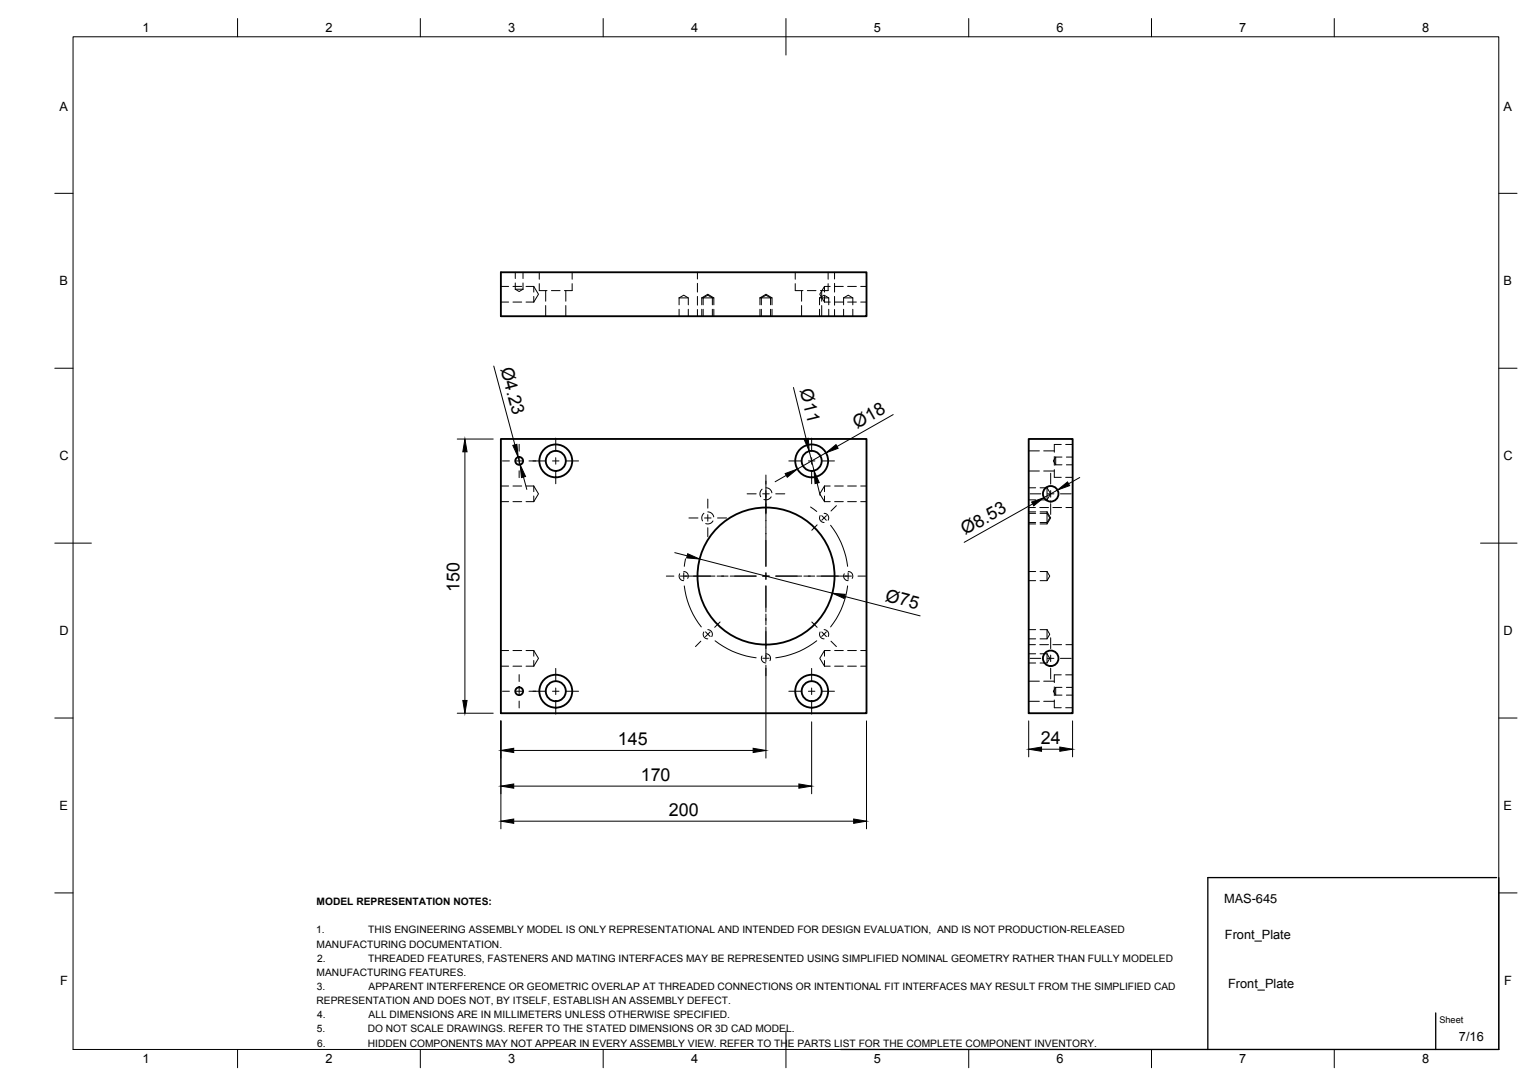
ISO-10303-21;
HEADER;
FILE_DESCRIPTION((''),'2;1');
FILE_NAME('Front_Plate.step','2026-10-09T10:54:55-07:00',(''),(''),'','','');
FILE_SCHEMA (('AUTOMOTIVE_DESIGN { 1 0 10303 214 3 1 1 }'));
ENDSEC;
DATA;
#10=MECHANICAL_DESIGN_GEOMETRIC_PRESENTATION_REPRESENTATION('',(#598),#63824);
#568=SHAPE_REPRESENTATION_RELATIONSHIP('SRR','None',#63882,#583) ;
#583=ADVANCED_BREP_SHAPE_REPRESENTATION('',(#613),#63812) ;
#598=STYLED_ITEM('',(#63963),#613) ;
#613=MANIFOLD_SOLID_BREP('Body1',#15497) ;
#695=FACE_BOUND('',#2596,.T.) ;
#696=FACE_BOUND('',#2600,.T.) ;
#697=FACE_BOUND('',#2604,.T.) ;
#698=FACE_BOUND('',#2608,.T.) ;
#699=FACE_BOUND('',#2629,.T.) ;
#700=FACE_BOUND('',#2630,.T.) ;
#701=FACE_BOUND('',#2633,.T.) ;
#702=FACE_BOUND('',#2634,.T.) ;
#703=FACE_BOUND('',#2637,.T.) ;
#704=FACE_BOUND('',#2638,.T.) ;
#705=FACE_BOUND('',#2639,.T.) ;
#706=FACE_BOUND('',#2640,.T.) ;
#707=FACE_BOUND('',#2641,.T.) ;
#708=FACE_BOUND('',#2642,.T.) ;
#709=FACE_BOUND('',#2643,.T.) ;
#710=FACE_BOUND('',#2645,.T.) ;
#711=FACE_BOUND('',#2646,.T.) ;
#712=FACE_BOUND('',#2647,.T.) ;
#713=FACE_BOUND('',#2648,.T.) ;
#714=FACE_BOUND('',#2649,.T.) ;
#715=FACE_BOUND('',#2650,.T.) ;
#716=FACE_BOUND('',#2651,.T.) ;
#717=FACE_BOUND('',#2652,.T.) ;
#718=FACE_BOUND('',#2653,.T.) ;
#719=FACE_BOUND('',#2654,.T.) ;
#720=FACE_BOUND('',#2655,.T.) ;
#721=FACE_BOUND('',#2656,.T.) ;
#722=FACE_BOUND('',#2657,.T.) ;
#866=PLANE('',#15917) ;
#867=PLANE('',#15924) ;
#868=PLANE('',#15931) ;
#869=PLANE('',#15938) ;
#870=PLANE('',#15980) ;
#871=PLANE('',#15981) ;
#872=PLANE('',#15982) ;
#873=PLANE('',#15983) ;
#874=PLANE('',#15984) ;
#875=PLANE('',#15985) ;
#1169=CYLINDRICAL_SURFACE('',#15895,2.117) ;
#1170=CYLINDRICAL_SURFACE('',#15899,2.117) ;
#1171=CYLINDRICAL_SURFACE('',#15903,4.263) ;
#1172=CYLINDRICAL_SURFACE('',#15907,4.263) ;
#1173=CYLINDRICAL_SURFACE('',#15911,4.263) ;
#1174=CYLINDRICAL_SURFACE('',#15915,4.263) ;
#1175=CYLINDRICAL_SURFACE('',#15920,9.) ;
#1176=CYLINDRICAL_SURFACE('',#15922,5.5) ;
#1177=CYLINDRICAL_SURFACE('',#15927,9.) ;
#1178=CYLINDRICAL_SURFACE('',#15929,5.5) ;
#1179=CYLINDRICAL_SURFACE('',#15934,9.) ;
#1180=CYLINDRICAL_SURFACE('',#15936,5.5) ;
#1181=CYLINDRICAL_SURFACE('',#15941,9.) ;
#1182=CYLINDRICAL_SURFACE('',#15943,5.5) ;
#1183=CYLINDRICAL_SURFACE('',#15947,3.3) ;
#1184=CYLINDRICAL_SURFACE('',#15951,2.5175) ;
#1185=CYLINDRICAL_SURFACE('',#15955,2.5175) ;
#1186=CYLINDRICAL_SURFACE('',#15959,2.5175) ;
#1187=CYLINDRICAL_SURFACE('',#15963,2.5175) ;
#1188=CYLINDRICAL_SURFACE('',#15967,2.5175) ;
#1189=CYLINDRICAL_SURFACE('',#15971,2.5175) ;
#1190=CYLINDRICAL_SURFACE('',#15975,3.3) ;
#1191=CYLINDRICAL_SURFACE('',#15977,37.5) ;
#1652=FACE_OUTER_BOUND('',#2583,.T.) ;
#1653=FACE_OUTER_BOUND('',#2584,.T.) ;
#1654=FACE_OUTER_BOUND('',#2585,.T.) ;
#1655=FACE_OUTER_BOUND('',#2586,.T.) ;
#1656=FACE_OUTER_BOUND('',#2587,.T.) ;
#1657=FACE_OUTER_BOUND('',#2588,.T.) ;
#1658=FACE_OUTER_BOUND('',#2589,.T.) ;
#1659=FACE_OUTER_BOUND('',#2590,.T.) ;
#1660=FACE_OUTER_BOUND('',#2591,.T.) ;
#1661=FACE_OUTER_BOUND('',#2592,.T.) ;
#1662=FACE_OUTER_BOUND('',#2593,.T.) ;
#1663=FACE_OUTER_BOUND('',#2594,.T.) ;
#1664=FACE_OUTER_BOUND('',#2595,.T.) ;
#1665=FACE_OUTER_BOUND('',#2597,.T.) ;
#1666=FACE_OUTER_BOUND('',#2598,.T.) ;
#1667=FACE_OUTER_BOUND('',#2599,.T.) ;
#1668=FACE_OUTER_BOUND('',#2601,.T.) ;
#1669=FACE_OUTER_BOUND('',#2602,.T.) ;
#1670=FACE_OUTER_BOUND('',#2603,.T.) ;
#1671=FACE_OUTER_BOUND('',#2605,.T.) ;
#1672=FACE_OUTER_BOUND('',#2606,.T.) ;
#1673=FACE_OUTER_BOUND('',#2607,.T.) ;
#1674=FACE_OUTER_BOUND('',#2609,.T.) ;
#1675=FACE_OUTER_BOUND('',#2610,.T.) ;
#1676=FACE_OUTER_BOUND('',#2611,.T.) ;
#1677=FACE_OUTER_BOUND('',#2612,.T.) ;
#1678=FACE_OUTER_BOUND('',#2613,.T.) ;
#1679=FACE_OUTER_BOUND('',#2614,.T.) ;
#1680=FACE_OUTER_BOUND('',#2615,.T.) ;
#1681=FACE_OUTER_BOUND('',#2616,.T.) ;
#1682=FACE_OUTER_BOUND('',#2617,.T.) ;
#1683=FACE_OUTER_BOUND('',#2618,.T.) ;
#1684=FACE_OUTER_BOUND('',#2619,.T.) ;
#1685=FACE_OUTER_BOUND('',#2620,.T.) ;
#1686=FACE_OUTER_BOUND('',#2621,.T.) ;
#1687=FACE_OUTER_BOUND('',#2622,.T.) ;
#1688=FACE_OUTER_BOUND('',#2623,.T.) ;
#1689=FACE_OUTER_BOUND('',#2624,.T.) ;
#1690=FACE_OUTER_BOUND('',#2625,.T.) ;
#1691=FACE_OUTER_BOUND('',#2626,.T.) ;
#1692=FACE_OUTER_BOUND('',#2627,.T.) ;
#1693=FACE_OUTER_BOUND('',#2628,.T.) ;
#1694=FACE_OUTER_BOUND('',#2631,.T.) ;
#1695=FACE_OUTER_BOUND('',#2632,.T.) ;
#1696=FACE_OUTER_BOUND('',#2635,.T.) ;
#1697=FACE_OUTER_BOUND('',#2636,.T.) ;
#1698=FACE_OUTER_BOUND('',#2644,.T.) ;
#2583=EDGE_LOOP('',(#10232,#10233,#10234)) ;
#2584=EDGE_LOOP('',(#10235,#10236,#10237,#10238)) ;
#2585=EDGE_LOOP('',(#10239,#10240,#10241)) ;
#2586=EDGE_LOOP('',(#10242,#10243,#10244,#10245)) ;
#2587=EDGE_LOOP('',(#10246,#10247,#10248)) ;
#2588=EDGE_LOOP('',(#10249,#10250,#10251,#10252)) ;
#2589=EDGE_LOOP('',(#10253,#10254,#10255)) ;
#2590=EDGE_LOOP('',(#10256,#10257,#10258,#10259)) ;
#2591=EDGE_LOOP('',(#10260,#10261,#10262)) ;
#2592=EDGE_LOOP('',(#10263,#10264,#10265,#10266)) ;
#2593=EDGE_LOOP('',(#10267,#10268,#10269)) ;
#2594=EDGE_LOOP('',(#10270,#10271,#10272,#10273)) ;
#2595=EDGE_LOOP('',(#10274)) ;
#2596=EDGE_LOOP('',(#10275)) ;
#2597=EDGE_LOOP('',(#10276,#10277,#10278,#10279)) ;
#2598=EDGE_LOOP('',(#10280,#10281,#10282,#10283)) ;
#2599=EDGE_LOOP('',(#10284)) ;
#2600=EDGE_LOOP('',(#10285)) ;
#2601=EDGE_LOOP('',(#10286,#10287,#10288,#10289)) ;
#2602=EDGE_LOOP('',(#10290,#10291,#10292,#10293)) ;
#2603=EDGE_LOOP('',(#10294)) ;
#2604=EDGE_LOOP('',(#10295)) ;
#2605=EDGE_LOOP('',(#10296,#10297,#10298,#10299)) ;
#2606=EDGE_LOOP('',(#10300,#10301,#10302,#10303)) ;
#2607=EDGE_LOOP('',(#10304)) ;
#2608=EDGE_LOOP('',(#10305)) ;
#2609=EDGE_LOOP('',(#10306,#10307,#10308,#10309)) ;
#2610=EDGE_LOOP('',(#10310,#10311,#10312,#10313)) ;
#2611=EDGE_LOOP('',(#10314,#10315,#10316)) ;
#2612=EDGE_LOOP('',(#10317,#10318,#10319,#10320)) ;
#2613=EDGE_LOOP('',(#10321,#10322,#10323)) ;
#2614=EDGE_LOOP('',(#10324,#10325,#10326,#10327)) ;
#2615=EDGE_LOOP('',(#10328,#10329,#10330)) ;
#2616=EDGE_LOOP('',(#10331,#10332,#10333,#10334)) ;
#2617=EDGE_LOOP('',(#10335,#10336,#10337)) ;
#2618=EDGE_LOOP('',(#10338,#10339,#10340,#10341)) ;
#2619=EDGE_LOOP('',(#10342,#10343,#10344)) ;
#2620=EDGE_LOOP('',(#10345,#10346,#10347,#10348)) ;
#2621=EDGE_LOOP('',(#10349,#10350,#10351)) ;
#2622=EDGE_LOOP('',(#10352,#10353,#10354,#10355)) ;
#2623=EDGE_LOOP('',(#10356,#10357,#10358)) ;
#2624=EDGE_LOOP('',(#10359,#10360,#10361,#10362)) ;
#2625=EDGE_LOOP('',(#10363,#10364,#10365)) ;
#2626=EDGE_LOOP('',(#10366,#10367,#10368,#10369)) ;
#2627=EDGE_LOOP('',(#10370,#10371,#10372,#10373)) ;
#2628=EDGE_LOOP('',(#10374,#10375,#10376,#10377)) ;
#2629=EDGE_LOOP('',(#10378)) ;
#2630=EDGE_LOOP('',(#10379)) ;
#2631=EDGE_LOOP('',(#10380,#10381,#10382,#10383)) ;
#2632=EDGE_LOOP('',(#10384,#10385,#10386,#10387)) ;
#2633=EDGE_LOOP('',(#10388)) ;
#2634=EDGE_LOOP('',(#10389)) ;
#2635=EDGE_LOOP('',(#10390,#10391,#10392,#10393)) ;
#2636=EDGE_LOOP('',(#10394,#10395,#10396,#10397)) ;
#2637=EDGE_LOOP('',(#10398)) ;
#2638=EDGE_LOOP('',(#10399)) ;
#2639=EDGE_LOOP('',(#10400)) ;
#2640=EDGE_LOOP('',(#10401)) ;
#2641=EDGE_LOOP('',(#10402)) ;
#2642=EDGE_LOOP('',(#10403)) ;
#2643=EDGE_LOOP('',(#10404)) ;
#2644=EDGE_LOOP('',(#10405,#10406,#10407,#10408)) ;
#2645=EDGE_LOOP('',(#10409)) ;
#2646=EDGE_LOOP('',(#10410)) ;
#2647=EDGE_LOOP('',(#10411)) ;
#2648=EDGE_LOOP('',(#10412)) ;
#2649=EDGE_LOOP('',(#10413)) ;
#2650=EDGE_LOOP('',(#10414)) ;
#2651=EDGE_LOOP('',(#10415)) ;
#2652=EDGE_LOOP('',(#10416)) ;
#2653=EDGE_LOOP('',(#10417)) ;
#2654=EDGE_LOOP('',(#10418)) ;
#2655=EDGE_LOOP('',(#10419)) ;
#2656=EDGE_LOOP('',(#10420)) ;
#2657=EDGE_LOOP('',(#10421)) ;
#3580=CIRCLE('',#15894,2.117) ;
#3581=CIRCLE('',#15896,2.117) ;
#3582=CIRCLE('',#15898,2.117) ;
#3583=CIRCLE('',#15900,2.117) ;
#3584=CIRCLE('',#15902,4.263) ;
#3585=CIRCLE('',#15904,4.263) ;
#3586=CIRCLE('',#15906,4.263) ;
#3587=CIRCLE('',#15908,4.263) ;
#3588=CIRCLE('',#15910,4.263) ;
#3589=CIRCLE('',#15912,4.263) ;
#3590=CIRCLE('',#15914,4.263) ;
#3591=CIRCLE('',#15916,4.263) ;
#3592=CIRCLE('',#15918,9.) ;
#3593=CIRCLE('',#15919,5.5) ;
#3594=CIRCLE('',#15921,9.) ;
#3595=CIRCLE('',#15923,5.5) ;
#3596=CIRCLE('',#15925,9.) ;
#3597=CIRCLE('',#15926,5.5) ;
#3598=CIRCLE('',#15928,9.) ;
#3599=CIRCLE('',#15930,5.5) ;
#3600=CIRCLE('',#15932,9.) ;
#3601=CIRCLE('',#15933,5.5) ;
#3602=CIRCLE('',#15935,9.) ;
#3603=CIRCLE('',#15937,5.5) ;
#3604=CIRCLE('',#15939,9.) ;
#3605=CIRCLE('',#15940,5.5) ;
#3606=CIRCLE('',#15942,9.) ;
#3607=CIRCLE('',#15944,5.5) ;
#3608=CIRCLE('',#15946,3.3) ;
#3609=CIRCLE('',#15948,3.3) ;
#3610=CIRCLE('',#15950,2.5175) ;
#3611=CIRCLE('',#15952,2.5175) ;
#3612=CIRCLE('',#15954,2.5175) ;
#3613=CIRCLE('',#15956,2.5175) ;
#3614=CIRCLE('',#15958,2.5175) ;
#3615=CIRCLE('',#15960,2.5175) ;
#3616=CIRCLE('',#15962,2.5175) ;
#3617=CIRCLE('',#15964,2.5175) ;
#3618=CIRCLE('',#15966,2.5175) ;
#3619=CIRCLE('',#15968,2.5175) ;
#3620=CIRCLE('',#15970,2.5175) ;
#3621=CIRCLE('',#15972,2.5175) ;
#3622=CIRCLE('',#15974,3.3) ;
#3623=CIRCLE('',#15976,3.3) ;
#3624=CIRCLE('',#15978,37.5) ;
#3625=CIRCLE('',#15979,37.5) ;
#4799=LINE('',#23492,#5455) ;
#4800=LINE('',#23497,#5456) ;
#4801=LINE('',#23501,#5457) ;
#4802=LINE('',#23506,#5458) ;
#4803=LINE('',#23510,#5459) ;
#4804=LINE('',#23515,#5460) ;
#4805=LINE('',#23519,#5461) ;
#4806=LINE('',#23524,#5462) ;
#4807=LINE('',#23528,#5463) ;
#4808=LINE('',#23533,#5464) ;
#4809=LINE('',#23537,#5465) ;
#4810=LINE('',#23542,#5466) ;
#4811=LINE('',#23550,#5467) ;
#4812=LINE('',#23555,#5468) ;
#4813=LINE('',#23563,#5469) ;
#4814=LINE('',#23568,#5470) ;
#4815=LINE('',#23576,#5471) ;
#4816=LINE('',#23581,#5472) ;
#4817=LINE('',#23589,#5473) ;
#4818=LINE('',#23594,#5474) ;
#4819=LINE('',#23598,#5475) ;
#4820=LINE('',#23602,#5476) ;
#4821=LINE('',#23607,#5477) ;
#4822=LINE('',#23611,#5478) ;
#4823=LINE('',#23616,#5479) ;
#4824=LINE('',#23620,#5480) ;
#4825=LINE('',#23625,#5481) ;
#4826=LINE('',#23629,#5482) ;
#4827=LINE('',#23634,#5483) ;
#4828=LINE('',#23638,#5484) ;
#4829=LINE('',#23643,#5485) ;
#4830=LINE('',#23647,#5486) ;
#4831=LINE('',#23652,#5487) ;
#4832=LINE('',#23656,#5488) ;
#4833=LINE('',#23661,#5489) ;
#4834=LINE('',#23665,#5490) ;
#4835=LINE('',#23671,#5491) ;
#4836=LINE('',#23676,#5492) ;
#4837=LINE('',#23678,#5493) ;
#4838=LINE('',#23680,#5494) ;
#4839=LINE('',#23681,#5495) ;
#4840=LINE('',#23684,#5496) ;
#4841=LINE('',#23686,#5497) ;
#4842=LINE('',#23687,#5498) ;
#4843=LINE('',#23690,#5499) ;
#4844=LINE('',#23692,#5500) ;
#4845=LINE('',#23693,#5501) ;
#4846=LINE('',#23695,#5502) ;
#4847=LINE('',#23696,#5503) ;
#5455=VECTOR('',#18449,1.20708774962173) ;
#5456=VECTOR('',#18456,2.117) ;
#5457=VECTOR('',#18459,1.20708774962173) ;
#5458=VECTOR('',#18466,2.117) ;
#5459=VECTOR('',#18469,2.42186816158307) ;
#5460=VECTOR('',#18476,4.263) ;
#5461=VECTOR('',#18479,2.42186816158307) ;
#5462=VECTOR('',#18486,4.263) ;
#5463=VECTOR('',#18489,2.42186816158307) ;
#5464=VECTOR('',#18496,4.263) ;
#5465=VECTOR('',#18499,2.42186816158307) ;
#5466=VECTOR('',#18506,4.263) ;
#5467=VECTOR('',#18515,9.) ;
#5468=VECTOR('',#18522,5.5) ;
#5469=VECTOR('',#18531,9.) ;
#5470=VECTOR('',#18538,5.5) ;
#5471=VECTOR('',#18547,9.) ;
#5472=VECTOR('',#18554,5.5) ;
#5473=VECTOR('',#18563,9.) ;
#5474=VECTOR('',#18570,5.5) ;
#5475=VECTOR('',#18573,1.65) ;
#5476=VECTOR('',#18578,3.3) ;
#5477=VECTOR('',#18583,1.44243074893998) ;
#5478=VECTOR('',#18588,2.5175) ;
#5479=VECTOR('',#18593,1.44243074893998) ;
#5480=VECTOR('',#18598,2.5175) ;
#5481=VECTOR('',#18603,1.44243074893998) ;
#5482=VECTOR('',#18608,2.5175) ;
#5483=VECTOR('',#18613,1.44243074893998) ;
#5484=VECTOR('',#18618,2.5175) ;
#5485=VECTOR('',#18623,1.44243074893998) ;
#5486=VECTOR('',#18628,2.5175) ;
#5487=VECTOR('',#18633,1.44243074893998) ;
#5488=VECTOR('',#18638,2.5175) ;
#5489=VECTOR('',#18643,1.65) ;
#5490=VECTOR('',#18648,3.3) ;
#5491=VECTOR('',#18655,37.5) ;
#5492=VECTOR('',#18660,10.) ;
#5493=VECTOR('',#18661,10.) ;
#5494=VECTOR('',#18662,10.) ;
#5495=VECTOR('',#18663,10.) ;
#5496=VECTOR('',#18666,10.) ;
#5497=VECTOR('',#18667,10.) ;
#5498=VECTOR('',#18668,10.) ;
#5499=VECTOR('',#18671,10.) ;
#5500=VECTOR('',#18672,10.) ;
#5501=VECTOR('',#18673,10.) ;
#5502=VECTOR('',#18676,10.) ;
#5503=VECTOR('',#18677,10.) ;
#6152=VERTEX_POINT('',#23490) ;
#6153=VERTEX_POINT('',#23491) ;
#6154=VERTEX_POINT('',#23495) ;
#6155=VERTEX_POINT('',#23499) ;
#6156=VERTEX_POINT('',#23500) ;
#6157=VERTEX_POINT('',#23504) ;
#6158=VERTEX_POINT('',#23508) ;
#6159=VERTEX_POINT('',#23509) ;
#6160=VERTEX_POINT('',#23513) ;
#6161=VERTEX_POINT('',#23517) ;
#6162=VERTEX_POINT('',#23518) ;
#6163=VERTEX_POINT('',#23522) ;
#6164=VERTEX_POINT('',#23526) ;
#6165=VERTEX_POINT('',#23527) ;
#6166=VERTEX_POINT('',#23531) ;
#6167=VERTEX_POINT('',#23535) ;
#6168=VERTEX_POINT('',#23536) ;
#6169=VERTEX_POINT('',#23540) ;
#6170=VERTEX_POINT('',#23544) ;
#6171=VERTEX_POINT('',#23546) ;
#6172=VERTEX_POINT('',#23549) ;
#6173=VERTEX_POINT('',#23553) ;
#6174=VERTEX_POINT('',#23557) ;
#6175=VERTEX_POINT('',#23559) ;
#6176=VERTEX_POINT('',#23562) ;
#6177=VERTEX_POINT('',#23566) ;
#6178=VERTEX_POINT('',#23570) ;
#6179=VERTEX_POINT('',#23572) ;
#6180=VERTEX_POINT('',#23575) ;
#6181=VERTEX_POINT('',#23579) ;
#6182=VERTEX_POINT('',#23583) ;
#6183=VERTEX_POINT('',#23585) ;
#6184=VERTEX_POINT('',#23588) ;
#6185=VERTEX_POINT('',#23592) ;
#6186=VERTEX_POINT('',#23596) ;
#6187=VERTEX_POINT('',#23597) ;
#6188=VERTEX_POINT('',#23601) ;
#6189=VERTEX_POINT('',#23605) ;
#6190=VERTEX_POINT('',#23606) ;
#6191=VERTEX_POINT('',#23610) ;
#6192=VERTEX_POINT('',#23614) ;
#6193=VERTEX_POINT('',#23615) ;
#6194=VERTEX_POINT('',#23619) ;
#6195=VERTEX_POINT('',#23623) ;
#6196=VERTEX_POINT('',#23624) ;
#6197=VERTEX_POINT('',#23628) ;
#6198=VERTEX_POINT('',#23632) ;
#6199=VERTEX_POINT('',#23633) ;
#6200=VERTEX_POINT('',#23637) ;
#6201=VERTEX_POINT('',#23641) ;
#6202=VERTEX_POINT('',#23642) ;
#6203=VERTEX_POINT('',#23646) ;
#6204=VERTEX_POINT('',#23650) ;
#6205=VERTEX_POINT('',#23651) ;
#6206=VERTEX_POINT('',#23655) ;
#6207=VERTEX_POINT('',#23659) ;
#6208=VERTEX_POINT('',#23660) ;
#6209=VERTEX_POINT('',#23664) ;
#6210=VERTEX_POINT('',#23668) ;
#6211=VERTEX_POINT('',#23670) ;
#6212=VERTEX_POINT('',#23674) ;
#6213=VERTEX_POINT('',#23675) ;
#6214=VERTEX_POINT('',#23677) ;
#6215=VERTEX_POINT('',#23679) ;
#6216=VERTEX_POINT('',#23683) ;
#6217=VERTEX_POINT('',#23685) ;
#6218=VERTEX_POINT('',#23689) ;
#6219=VERTEX_POINT('',#23691) ;
#7670=EDGE_CURVE('',#6152,#6153,#4799,.T.) ;
#7671=EDGE_CURVE('',#6153,#6153,#3580,.T.) ;
#7672=EDGE_CURVE('',#6154,#6154,#3581,.T.) ;
#7673=EDGE_CURVE('',#6154,#6153,#4800,.T.) ;
#7674=EDGE_CURVE('',#6155,#6156,#4801,.T.) ;
#7675=EDGE_CURVE('',#6156,#6156,#3582,.T.) ;
#7676=EDGE_CURVE('',#6157,#6157,#3583,.T.) ;
#7677=EDGE_CURVE('',#6157,#6156,#4802,.T.) ;
#7678=EDGE_CURVE('',#6158,#6159,#4803,.T.) ;
#7679=EDGE_CURVE('',#6159,#6159,#3584,.T.) ;
#7680=EDGE_CURVE('',#6160,#6160,#3585,.T.) ;
#7681=EDGE_CURVE('',#6160,#6159,#4804,.T.) ;
#7682=EDGE_CURVE('',#6161,#6162,#4805,.T.) ;
#7683=EDGE_CURVE('',#6162,#6162,#3586,.T.) ;
#7684=EDGE_CURVE('',#6163,#6163,#3587,.T.) ;
#7685=EDGE_CURVE('',#6163,#6162,#4806,.T.) ;
#7686=EDGE_CURVE('',#6164,#6165,#4807,.T.) ;
#7687=EDGE_CURVE('',#6165,#6165,#3588,.T.) ;
#7688=EDGE_CURVE('',#6166,#6166,#3589,.T.) ;
#7689=EDGE_CURVE('',#6166,#6165,#4808,.T.) ;
#7690=EDGE_CURVE('',#6167,#6168,#4809,.T.) ;
#7691=EDGE_CURVE('',#6168,#6168,#3590,.T.) ;
#7692=EDGE_CURVE('',#6169,#6169,#3591,.T.) ;
#7693=EDGE_CURVE('',#6169,#6168,#4810,.T.) ;
#7694=EDGE_CURVE('',#6170,#6170,#3592,.T.) ;
#7695=EDGE_CURVE('',#6171,#6171,#3593,.T.) ;
#7696=EDGE_CURVE('',#6170,#6172,#4811,.T.) ;
#7697=EDGE_CURVE('',#6172,#6172,#3594,.T.) ;
#7698=EDGE_CURVE('',#6173,#6173,#3595,.T.) ;
#7699=EDGE_CURVE('',#6173,#6171,#4812,.T.) ;
#7700=EDGE_CURVE('',#6174,#6174,#3596,.T.) ;
#7701=EDGE_CURVE('',#6175,#6175,#3597,.T.) ;
#7702=EDGE_CURVE('',#6174,#6176,#4813,.T.) ;
#7703=EDGE_CURVE('',#6176,#6176,#3598,.T.) ;
#7704=EDGE_CURVE('',#6177,#6177,#3599,.T.) ;
#7705=EDGE_CURVE('',#6177,#6175,#4814,.T.) ;
#7706=EDGE_CURVE('',#6178,#6178,#3600,.T.) ;
#7707=EDGE_CURVE('',#6179,#6179,#3601,.T.) ;
#7708=EDGE_CURVE('',#6178,#6180,#4815,.T.) ;
#7709=EDGE_CURVE('',#6180,#6180,#3602,.T.) ;
#7710=EDGE_CURVE('',#6181,#6181,#3603,.T.) ;
#7711=EDGE_CURVE('',#6181,#6179,#4816,.T.) ;
#7712=EDGE_CURVE('',#6182,#6182,#3604,.T.) ;
#7713=EDGE_CURVE('',#6183,#6183,#3605,.T.) ;
#7714=EDGE_CURVE('',#6182,#6184,#4817,.T.) ;
#7715=EDGE_CURVE('',#6184,#6184,#3606,.T.) ;
#7716=EDGE_CURVE('',#6185,#6185,#3607,.T.) ;
#7717=EDGE_CURVE('',#6185,#6183,#4818,.T.) ;
#7718=EDGE_CURVE('',#6186,#6187,#4819,.T.) ;
#7719=EDGE_CURVE('',#6187,#6187,#3608,.T.) ;
#7720=EDGE_CURVE('',#6187,#6188,#4820,.T.) ;
#7721=EDGE_CURVE('',#6188,#6188,#3609,.T.) ;
#7722=EDGE_CURVE('',#6189,#6190,#4821,.T.) ;
#7723=EDGE_CURVE('',#6190,#6190,#3610,.T.) ;
#7724=EDGE_CURVE('',#6190,#6191,#4822,.T.) ;
#7725=EDGE_CURVE('',#6191,#6191,#3611,.F.) ;
#7726=EDGE_CURVE('',#6192,#6193,#4823,.T.) ;
#7727=EDGE_CURVE('',#6193,#6193,#3612,.T.) ;
#7728=EDGE_CURVE('',#6193,#6194,#4824,.T.) ;
#7729=EDGE_CURVE('',#6194,#6194,#3613,.F.) ;
#7730=EDGE_CURVE('',#6195,#6196,#4825,.T.) ;
#7731=EDGE_CURVE('',#6196,#6196,#3614,.T.) ;
#7732=EDGE_CURVE('',#6196,#6197,#4826,.T.) ;
#7733=EDGE_CURVE('',#6197,#6197,#3615,.F.) ;
#7734=EDGE_CURVE('',#6198,#6199,#4827,.T.) ;
#7735=EDGE_CURVE('',#6199,#6199,#3616,.T.) ;
#7736=EDGE_CURVE('',#6199,#6200,#4828,.T.) ;
#7737=EDGE_CURVE('',#6200,#6200,#3617,.F.) ;
#7738=EDGE_CURVE('',#6201,#6202,#4829,.T.) ;
#7739=EDGE_CURVE('',#6202,#6202,#3618,.T.) ;
#7740=EDGE_CURVE('',#6202,#6203,#4830,.T.) ;
#7741=EDGE_CURVE('',#6203,#6203,#3619,.F.) ;
#7742=EDGE_CURVE('',#6204,#6205,#4831,.T.) ;
#7743=EDGE_CURVE('',#6205,#6205,#3620,.T.) ;
#7744=EDGE_CURVE('',#6205,#6206,#4832,.T.) ;
#7745=EDGE_CURVE('',#6206,#6206,#3621,.F.) ;
#7746=EDGE_CURVE('',#6207,#6208,#4833,.T.) ;
#7747=EDGE_CURVE('',#6208,#6208,#3622,.T.) ;
#7748=EDGE_CURVE('',#6208,#6209,#4834,.T.) ;
#7749=EDGE_CURVE('',#6209,#6209,#3623,.T.) ;
#7750=EDGE_CURVE('',#6210,#6210,#3624,.T.) ;
#7751=EDGE_CURVE('',#6210,#6211,#4835,.T.) ;
#7752=EDGE_CURVE('',#6211,#6211,#3625,.T.) ;
#7753=EDGE_CURVE('',#6212,#6213,#4836,.T.) ;
#7754=EDGE_CURVE('',#6213,#6214,#4837,.T.) ;
#7755=EDGE_CURVE('',#6214,#6215,#4838,.T.) ;
#7756=EDGE_CURVE('',#6212,#6215,#4839,.T.) ;
#7757=EDGE_CURVE('',#6213,#6216,#4840,.T.) ;
#7758=EDGE_CURVE('',#6216,#6217,#4841,.T.) ;
#7759=EDGE_CURVE('',#6217,#6214,#4842,.T.) ;
#7760=EDGE_CURVE('',#6218,#6216,#4843,.T.) ;
#7761=EDGE_CURVE('',#6218,#6219,#4844,.T.) ;
#7762=EDGE_CURVE('',#6219,#6217,#4845,.T.) ;
#7763=EDGE_CURVE('',#6218,#6212,#4846,.T.) ;
#7764=EDGE_CURVE('',#6215,#6219,#4847,.T.) ;
#10232=ORIENTED_EDGE('',*,*,#7670,.T.) ;
#10233=ORIENTED_EDGE('',*,*,#7671,.F.) ;
#10234=ORIENTED_EDGE('',*,*,#7670,.F.) ;
#10235=ORIENTED_EDGE('',*,*,#7672,.F.) ;
#10236=ORIENTED_EDGE('',*,*,#7673,.T.) ;
#10237=ORIENTED_EDGE('',*,*,#7671,.T.) ;
#10238=ORIENTED_EDGE('',*,*,#7673,.F.) ;
#10239=ORIENTED_EDGE('',*,*,#7674,.T.) ;
#10240=ORIENTED_EDGE('',*,*,#7675,.F.) ;
#10241=ORIENTED_EDGE('',*,*,#7674,.F.) ;
#10242=ORIENTED_EDGE('',*,*,#7676,.F.) ;
#10243=ORIENTED_EDGE('',*,*,#7677,.T.) ;
#10244=ORIENTED_EDGE('',*,*,#7675,.T.) ;
#10245=ORIENTED_EDGE('',*,*,#7677,.F.) ;
#10246=ORIENTED_EDGE('',*,*,#7678,.T.) ;
#10247=ORIENTED_EDGE('',*,*,#7679,.F.) ;
#10248=ORIENTED_EDGE('',*,*,#7678,.F.) ;
#10249=ORIENTED_EDGE('',*,*,#7680,.F.) ;
#10250=ORIENTED_EDGE('',*,*,#7681,.T.) ;
#10251=ORIENTED_EDGE('',*,*,#7679,.T.) ;
#10252=ORIENTED_EDGE('',*,*,#7681,.F.) ;
#10253=ORIENTED_EDGE('',*,*,#7682,.T.) ;
#10254=ORIENTED_EDGE('',*,*,#7683,.F.) ;
#10255=ORIENTED_EDGE('',*,*,#7682,.F.) ;
#10256=ORIENTED_EDGE('',*,*,#7684,.F.) ;
#10257=ORIENTED_EDGE('',*,*,#7685,.T.) ;
#10258=ORIENTED_EDGE('',*,*,#7683,.T.) ;
#10259=ORIENTED_EDGE('',*,*,#7685,.F.) ;
#10260=ORIENTED_EDGE('',*,*,#7686,.T.) ;
#10261=ORIENTED_EDGE('',*,*,#7687,.F.) ;
#10262=ORIENTED_EDGE('',*,*,#7686,.F.) ;
#10263=ORIENTED_EDGE('',*,*,#7688,.F.) ;
#10264=ORIENTED_EDGE('',*,*,#7689,.T.) ;
#10265=ORIENTED_EDGE('',*,*,#7687,.T.) ;
#10266=ORIENTED_EDGE('',*,*,#7689,.F.) ;
#10267=ORIENTED_EDGE('',*,*,#7690,.T.) ;
#10268=ORIENTED_EDGE('',*,*,#7691,.F.) ;
#10269=ORIENTED_EDGE('',*,*,#7690,.F.) ;
#10270=ORIENTED_EDGE('',*,*,#7692,.F.) ;
#10271=ORIENTED_EDGE('',*,*,#7693,.T.) ;
#10272=ORIENTED_EDGE('',*,*,#7691,.T.) ;
#10273=ORIENTED_EDGE('',*,*,#7693,.F.) ;
#10274=ORIENTED_EDGE('',*,*,#7694,.T.) ;
#10275=ORIENTED_EDGE('',*,*,#7695,.F.) ;
#10276=ORIENTED_EDGE('',*,*,#7694,.F.) ;
#10277=ORIENTED_EDGE('',*,*,#7696,.T.) ;
#10278=ORIENTED_EDGE('',*,*,#7697,.T.) ;
#10279=ORIENTED_EDGE('',*,*,#7696,.F.) ;
#10280=ORIENTED_EDGE('',*,*,#7698,.T.) ;
#10281=ORIENTED_EDGE('',*,*,#7699,.T.) ;
#10282=ORIENTED_EDGE('',*,*,#7695,.T.) ;
#10283=ORIENTED_EDGE('',*,*,#7699,.F.) ;
#10284=ORIENTED_EDGE('',*,*,#7700,.T.) ;
#10285=ORIENTED_EDGE('',*,*,#7701,.F.) ;
#10286=ORIENTED_EDGE('',*,*,#7700,.F.) ;
#10287=ORIENTED_EDGE('',*,*,#7702,.T.) ;
#10288=ORIENTED_EDGE('',*,*,#7703,.T.) ;
#10289=ORIENTED_EDGE('',*,*,#7702,.F.) ;
#10290=ORIENTED_EDGE('',*,*,#7704,.T.) ;
#10291=ORIENTED_EDGE('',*,*,#7705,.T.) ;
#10292=ORIENTED_EDGE('',*,*,#7701,.T.) ;
#10293=ORIENTED_EDGE('',*,*,#7705,.F.) ;
#10294=ORIENTED_EDGE('',*,*,#7706,.T.) ;
#10295=ORIENTED_EDGE('',*,*,#7707,.F.) ;
#10296=ORIENTED_EDGE('',*,*,#7706,.F.) ;
#10297=ORIENTED_EDGE('',*,*,#7708,.T.) ;
#10298=ORIENTED_EDGE('',*,*,#7709,.T.) ;
#10299=ORIENTED_EDGE('',*,*,#7708,.F.) ;
#10300=ORIENTED_EDGE('',*,*,#7710,.T.) ;
#10301=ORIENTED_EDGE('',*,*,#7711,.T.) ;
#10302=ORIENTED_EDGE('',*,*,#7707,.T.) ;
#10303=ORIENTED_EDGE('',*,*,#7711,.F.) ;
#10304=ORIENTED_EDGE('',*,*,#7712,.T.) ;
#10305=ORIENTED_EDGE('',*,*,#7713,.F.) ;
#10306=ORIENTED_EDGE('',*,*,#7712,.F.) ;
#10307=ORIENTED_EDGE('',*,*,#7714,.T.) ;
#10308=ORIENTED_EDGE('',*,*,#7715,.T.) ;
#10309=ORIENTED_EDGE('',*,*,#7714,.F.) ;
#10310=ORIENTED_EDGE('',*,*,#7716,.T.) ;
#10311=ORIENTED_EDGE('',*,*,#7717,.T.) ;
#10312=ORIENTED_EDGE('',*,*,#7713,.T.) ;
#10313=ORIENTED_EDGE('',*,*,#7717,.F.) ;
#10314=ORIENTED_EDGE('',*,*,#7718,.T.) ;
#10315=ORIENTED_EDGE('',*,*,#7719,.T.) ;
#10316=ORIENTED_EDGE('',*,*,#7718,.F.) ;
#10317=ORIENTED_EDGE('',*,*,#7719,.F.) ;
#10318=ORIENTED_EDGE('',*,*,#7720,.T.) ;
#10319=ORIENTED_EDGE('',*,*,#7721,.T.) ;
#10320=ORIENTED_EDGE('',*,*,#7720,.F.) ;
#10321=ORIENTED_EDGE('',*,*,#7722,.T.) ;
#10322=ORIENTED_EDGE('',*,*,#7723,.T.) ;
#10323=ORIENTED_EDGE('',*,*,#7722,.F.) ;
#10324=ORIENTED_EDGE('',*,*,#7723,.F.) ;
#10325=ORIENTED_EDGE('',*,*,#7724,.T.) ;
#10326=ORIENTED_EDGE('',*,*,#7725,.T.) ;
#10327=ORIENTED_EDGE('',*,*,#7724,.F.) ;
#10328=ORIENTED_EDGE('',*,*,#7726,.T.) ;
#10329=ORIENTED_EDGE('',*,*,#7727,.T.) ;
#10330=ORIENTED_EDGE('',*,*,#7726,.F.) ;
#10331=ORIENTED_EDGE('',*,*,#7727,.F.) ;
#10332=ORIENTED_EDGE('',*,*,#7728,.T.) ;
#10333=ORIENTED_EDGE('',*,*,#7729,.T.) ;
#10334=ORIENTED_EDGE('',*,*,#7728,.F.) ;
#10335=ORIENTED_EDGE('',*,*,#7730,.T.) ;
#10336=ORIENTED_EDGE('',*,*,#7731,.T.) ;
#10337=ORIENTED_EDGE('',*,*,#7730,.F.) ;
#10338=ORIENTED_EDGE('',*,*,#7731,.F.) ;
#10339=ORIENTED_EDGE('',*,*,#7732,.T.) ;
#10340=ORIENTED_EDGE('',*,*,#7733,.T.) ;
#10341=ORIENTED_EDGE('',*,*,#7732,.F.) ;
#10342=ORIENTED_EDGE('',*,*,#7734,.T.) ;
#10343=ORIENTED_EDGE('',*,*,#7735,.T.) ;
#10344=ORIENTED_EDGE('',*,*,#7734,.F.) ;
#10345=ORIENTED_EDGE('',*,*,#7735,.F.) ;
#10346=ORIENTED_EDGE('',*,*,#7736,.T.) ;
#10347=ORIENTED_EDGE('',*,*,#7737,.T.) ;
#10348=ORIENTED_EDGE('',*,*,#7736,.F.) ;
#10349=ORIENTED_EDGE('',*,*,#7738,.T.) ;
#10350=ORIENTED_EDGE('',*,*,#7739,.T.) ;
#10351=ORIENTED_EDGE('',*,*,#7738,.F.) ;
#10352=ORIENTED_EDGE('',*,*,#7739,.F.) ;
#10353=ORIENTED_EDGE('',*,*,#7740,.T.) ;
#10354=ORIENTED_EDGE('',*,*,#7741,.T.) ;
#10355=ORIENTED_EDGE('',*,*,#7740,.F.) ;
#10356=ORIENTED_EDGE('',*,*,#7742,.T.) ;
#10357=ORIENTED_EDGE('',*,*,#7743,.T.) ;
#10358=ORIENTED_EDGE('',*,*,#7742,.F.) ;
#10359=ORIENTED_EDGE('',*,*,#7743,.F.) ;
#10360=ORIENTED_EDGE('',*,*,#7744,.T.) ;
#10361=ORIENTED_EDGE('',*,*,#7745,.T.) ;
#10362=ORIENTED_EDGE('',*,*,#7744,.F.) ;
#10363=ORIENTED_EDGE('',*,*,#7746,.T.) ;
#10364=ORIENTED_EDGE('',*,*,#7747,.T.) ;
#10365=ORIENTED_EDGE('',*,*,#7746,.F.) ;
#10366=ORIENTED_EDGE('',*,*,#7747,.F.) ;
#10367=ORIENTED_EDGE('',*,*,#7748,.T.) ;
#10368=ORIENTED_EDGE('',*,*,#7749,.T.) ;
#10369=ORIENTED_EDGE('',*,*,#7748,.F.) ;
#10370=ORIENTED_EDGE('',*,*,#7750,.T.) ;
#10371=ORIENTED_EDGE('',*,*,#7751,.T.) ;
#10372=ORIENTED_EDGE('',*,*,#7752,.T.) ;
#10373=ORIENTED_EDGE('',*,*,#7751,.F.) ;
#10374=ORIENTED_EDGE('',*,*,#7753,.T.) ;
#10375=ORIENTED_EDGE('',*,*,#7754,.T.) ;
#10376=ORIENTED_EDGE('',*,*,#7755,.T.) ;
#10377=ORIENTED_EDGE('',*,*,#7756,.F.) ;
#10378=ORIENTED_EDGE('',*,*,#7688,.T.) ;
#10379=ORIENTED_EDGE('',*,*,#7692,.T.) ;
#10380=ORIENTED_EDGE('',*,*,#7757,.T.) ;
#10381=ORIENTED_EDGE('',*,*,#7758,.T.) ;
#10382=ORIENTED_EDGE('',*,*,#7759,.T.) ;
#10383=ORIENTED_EDGE('',*,*,#7754,.F.) ;
#10384=ORIENTED_EDGE('',*,*,#7760,.F.) ;
#10385=ORIENTED_EDGE('',*,*,#7761,.T.) ;
#10386=ORIENTED_EDGE('',*,*,#7762,.T.) ;
#10387=ORIENTED_EDGE('',*,*,#7758,.F.) ;
#10388=ORIENTED_EDGE('',*,*,#7680,.T.) ;
#10389=ORIENTED_EDGE('',*,*,#7684,.T.) ;
#10390=ORIENTED_EDGE('',*,*,#7763,.T.) ;
#10391=ORIENTED_EDGE('',*,*,#7756,.T.) ;
#10392=ORIENTED_EDGE('',*,*,#7764,.T.) ;
#10393=ORIENTED_EDGE('',*,*,#7761,.F.) ;
#10394=ORIENTED_EDGE('',*,*,#7763,.F.) ;
#10395=ORIENTED_EDGE('',*,*,#7760,.T.) ;
#10396=ORIENTED_EDGE('',*,*,#7757,.F.) ;
#10397=ORIENTED_EDGE('',*,*,#7753,.F.) ;
#10398=ORIENTED_EDGE('',*,*,#7672,.T.) ;
#10399=ORIENTED_EDGE('',*,*,#7676,.T.) ;
#10400=ORIENTED_EDGE('',*,*,#7697,.F.) ;
#10401=ORIENTED_EDGE('',*,*,#7703,.F.) ;
#10402=ORIENTED_EDGE('',*,*,#7709,.F.) ;
#10403=ORIENTED_EDGE('',*,*,#7715,.F.) ;
#10404=ORIENTED_EDGE('',*,*,#7752,.F.) ;
#10405=ORIENTED_EDGE('',*,*,#7764,.F.) ;
#10406=ORIENTED_EDGE('',*,*,#7755,.F.) ;
#10407=ORIENTED_EDGE('',*,*,#7759,.F.) ;
#10408=ORIENTED_EDGE('',*,*,#7762,.F.) ;
#10409=ORIENTED_EDGE('',*,*,#7698,.F.) ;
#10410=ORIENTED_EDGE('',*,*,#7704,.F.) ;
#10411=ORIENTED_EDGE('',*,*,#7710,.F.) ;
#10412=ORIENTED_EDGE('',*,*,#7716,.F.) ;
#10413=ORIENTED_EDGE('',*,*,#7721,.F.) ;
#10414=ORIENTED_EDGE('',*,*,#7725,.F.) ;
#10415=ORIENTED_EDGE('',*,*,#7729,.F.) ;
#10416=ORIENTED_EDGE('',*,*,#7733,.F.) ;
#10417=ORIENTED_EDGE('',*,*,#7737,.F.) ;
#10418=ORIENTED_EDGE('',*,*,#7741,.F.) ;
#10419=ORIENTED_EDGE('',*,*,#7745,.F.) ;
#10420=ORIENTED_EDGE('',*,*,#7749,.F.) ;
#10421=ORIENTED_EDGE('',*,*,#7750,.F.) ;
#14516=CONICAL_SURFACE('',#15893,1.20708774962173,1.02974425867665) ;
#14517=CONICAL_SURFACE('',#15897,1.20708774962173,1.02974425867665) ;
#14518=CONICAL_SURFACE('',#15901,2.42186816158307,1.02974425867665) ;
#14519=CONICAL_SURFACE('',#15905,2.42186816158307,1.02974425867665) ;
#14520=CONICAL_SURFACE('',#15909,2.42186816158307,1.02974425867665) ;
#14521=CONICAL_SURFACE('',#15913,2.42186816158307,1.02974425867665) ;
#14522=CONICAL_SURFACE('',#15945,1.65,1.02974425867665) ;
#14523=CONICAL_SURFACE('',#15949,1.44243074893998,1.02974425867665) ;
#14524=CONICAL_SURFACE('',#15953,1.44243074893998,1.02974425867665) ;
#14525=CONICAL_SURFACE('',#15957,1.44243074893998,1.02974425867665) ;
#14526=CONICAL_SURFACE('',#15961,1.44243074893998,1.02974425867665) ;
#14527=CONICAL_SURFACE('',#15965,1.44243074893998,1.02974425867665) ;
#14528=CONICAL_SURFACE('',#15969,1.44243074893998,1.02974425867665) ;
#14529=CONICAL_SURFACE('',#15973,1.65,1.02974425867665) ;
#14740=ADVANCED_FACE('',(#1652),#14516,.F.) ;
#14741=ADVANCED_FACE('',(#1653),#1169,.F.) ;
#14742=ADVANCED_FACE('',(#1654),#14517,.F.) ;
#14743=ADVANCED_FACE('',(#1655),#1170,.F.) ;
#14744=ADVANCED_FACE('',(#1656),#14518,.F.) ;
#14745=ADVANCED_FACE('',(#1657),#1171,.F.) ;
#14746=ADVANCED_FACE('',(#1658),#14519,.F.) ;
#14747=ADVANCED_FACE('',(#1659),#1172,.F.) ;
#14748=ADVANCED_FACE('',(#1660),#14520,.F.) ;
#14749=ADVANCED_FACE('',(#1661),#1173,.F.) ;
#14750=ADVANCED_FACE('',(#1662),#14521,.F.) ;
#14751=ADVANCED_FACE('',(#1663),#1174,.F.) ;
#14752=ADVANCED_FACE('',(#1664,#695),#866,.T.) ;
#14753=ADVANCED_FACE('',(#1665),#1175,.F.) ;
#14754=ADVANCED_FACE('',(#1666),#1176,.F.) ;
#14755=ADVANCED_FACE('',(#1667,#696),#867,.T.) ;
#14756=ADVANCED_FACE('',(#1668),#1177,.F.) ;
#14757=ADVANCED_FACE('',(#1669),#1178,.F.) ;
#14758=ADVANCED_FACE('',(#1670,#697),#868,.T.) ;
#14759=ADVANCED_FACE('',(#1671),#1179,.F.) ;
#14760=ADVANCED_FACE('',(#1672),#1180,.F.) ;
#14761=ADVANCED_FACE('',(#1673,#698),#869,.T.) ;
#14762=ADVANCED_FACE('',(#1674),#1181,.F.) ;
#14763=ADVANCED_FACE('',(#1675),#1182,.F.) ;
#14764=ADVANCED_FACE('',(#1676),#14522,.F.) ;
#14765=ADVANCED_FACE('',(#1677),#1183,.F.) ;
#14766=ADVANCED_FACE('',(#1678),#14523,.F.) ;
#14767=ADVANCED_FACE('',(#1679),#1184,.F.) ;
#14768=ADVANCED_FACE('',(#1680),#14524,.F.) ;
#14769=ADVANCED_FACE('',(#1681),#1185,.F.) ;
#14770=ADVANCED_FACE('',(#1682),#14525,.F.) ;
#14771=ADVANCED_FACE('',(#1683),#1186,.F.) ;
#14772=ADVANCED_FACE('',(#1684),#14526,.F.) ;
#14773=ADVANCED_FACE('',(#1685),#1187,.F.) ;
#14774=ADVANCED_FACE('',(#1686),#14527,.F.) ;
#14775=ADVANCED_FACE('',(#1687),#1188,.F.) ;
#14776=ADVANCED_FACE('',(#1688),#14528,.F.) ;
#14777=ADVANCED_FACE('',(#1689),#1189,.F.) ;
#14778=ADVANCED_FACE('',(#1690),#14529,.F.) ;
#14779=ADVANCED_FACE('',(#1691),#1190,.F.) ;
#14780=ADVANCED_FACE('',(#1692),#1191,.F.) ;
#14781=ADVANCED_FACE('',(#1693,#699,#700),#870,.F.) ;
#14782=ADVANCED_FACE('',(#1694),#871,.F.) ;
#14783=ADVANCED_FACE('',(#1695,#701,#702),#872,.F.) ;
#14784=ADVANCED_FACE('',(#1696),#873,.F.) ;
#14785=ADVANCED_FACE('',(#1697,#703,#704,#705,#706,#707,#708,#709),#874,
 .F.) ;
#14786=ADVANCED_FACE('',(#1698,#710,#711,#712,#713,#714,#715,#716,#717,
#718,#719,#720,#721,#722),#875,.T.) ;
#15497=CLOSED_SHELL('',(#14740,#14741,#14742,#14743,#14744,#14745,#14746,
#14747,#14748,#14749,#14750,#14751,#14752,#14753,#14754,#14755,#14756,#14757,
#14758,#14759,#14760,#14761,#14762,#14763,#14764,#14765,#14766,#14767,#14768,
#14769,#14770,#14771,#14772,#14773,#14774,#14775,#14776,#14777,#14778,#14779,
#14780,#14781,#14782,#14783,#14784,#14785,#14786)) ;
#15892=AXIS2_PLACEMENT_3D('',#23488,#18445,#18446) ;
#15893=AXIS2_PLACEMENT_3D('',#23489,#18447,#18448) ;
#15894=AXIS2_PLACEMENT_3D('',#23493,#18450,#18451) ;
#15895=AXIS2_PLACEMENT_3D('',#23494,#18452,#18453) ;
#15896=AXIS2_PLACEMENT_3D('',#23496,#18454,#18455) ;
#15897=AXIS2_PLACEMENT_3D('',#23498,#18457,#18458) ;
#15898=AXIS2_PLACEMENT_3D('',#23502,#18460,#18461) ;
#15899=AXIS2_PLACEMENT_3D('',#23503,#18462,#18463) ;
#15900=AXIS2_PLACEMENT_3D('',#23505,#18464,#18465) ;
#15901=AXIS2_PLACEMENT_3D('',#23507,#18467,#18468) ;
#15902=AXIS2_PLACEMENT_3D('',#23511,#18470,#18471) ;
#15903=AXIS2_PLACEMENT_3D('',#23512,#18472,#18473) ;
#15904=AXIS2_PLACEMENT_3D('',#23514,#18474,#18475) ;
#15905=AXIS2_PLACEMENT_3D('',#23516,#18477,#18478) ;
#15906=AXIS2_PLACEMENT_3D('',#23520,#18480,#18481) ;
#15907=AXIS2_PLACEMENT_3D('',#23521,#18482,#18483) ;
#15908=AXIS2_PLACEMENT_3D('',#23523,#18484,#18485) ;
#15909=AXIS2_PLACEMENT_3D('',#23525,#18487,#18488) ;
#15910=AXIS2_PLACEMENT_3D('',#23529,#18490,#18491) ;
#15911=AXIS2_PLACEMENT_3D('',#23530,#18492,#18493) ;
#15912=AXIS2_PLACEMENT_3D('',#23532,#18494,#18495) ;
#15913=AXIS2_PLACEMENT_3D('',#23534,#18497,#18498) ;
#15914=AXIS2_PLACEMENT_3D('',#23538,#18500,#18501) ;
#15915=AXIS2_PLACEMENT_3D('',#23539,#18502,#18503) ;
#15916=AXIS2_PLACEMENT_3D('',#23541,#18504,#18505) ;
#15917=AXIS2_PLACEMENT_3D('',#23543,#18507,#18508) ;
#15918=AXIS2_PLACEMENT_3D('',#23545,#18509,#18510) ;
#15919=AXIS2_PLACEMENT_3D('',#23547,#18511,#18512) ;
#15920=AXIS2_PLACEMENT_3D('',#23548,#18513,#18514) ;
#15921=AXIS2_PLACEMENT_3D('',#23551,#18516,#18517) ;
#15922=AXIS2_PLACEMENT_3D('',#23552,#18518,#18519) ;
#15923=AXIS2_PLACEMENT_3D('',#23554,#18520,#18521) ;
#15924=AXIS2_PLACEMENT_3D('',#23556,#18523,#18524) ;
#15925=AXIS2_PLACEMENT_3D('',#23558,#18525,#18526) ;
#15926=AXIS2_PLACEMENT_3D('',#23560,#18527,#18528) ;
#15927=AXIS2_PLACEMENT_3D('',#23561,#18529,#18530) ;
#15928=AXIS2_PLACEMENT_3D('',#23564,#18532,#18533) ;
#15929=AXIS2_PLACEMENT_3D('',#23565,#18534,#18535) ;
#15930=AXIS2_PLACEMENT_3D('',#23567,#18536,#18537) ;
#15931=AXIS2_PLACEMENT_3D('',#23569,#18539,#18540) ;
#15932=AXIS2_PLACEMENT_3D('',#23571,#18541,#18542) ;
#15933=AXIS2_PLACEMENT_3D('',#23573,#18543,#18544) ;
#15934=AXIS2_PLACEMENT_3D('',#23574,#18545,#18546) ;
#15935=AXIS2_PLACEMENT_3D('',#23577,#18548,#18549) ;
#15936=AXIS2_PLACEMENT_3D('',#23578,#18550,#18551) ;
#15937=AXIS2_PLACEMENT_3D('',#23580,#18552,#18553) ;
#15938=AXIS2_PLACEMENT_3D('',#23582,#18555,#18556) ;
#15939=AXIS2_PLACEMENT_3D('',#23584,#18557,#18558) ;
#15940=AXIS2_PLACEMENT_3D('',#23586,#18559,#18560) ;
#15941=AXIS2_PLACEMENT_3D('',#23587,#18561,#18562) ;
#15942=AXIS2_PLACEMENT_3D('',#23590,#18564,#18565) ;
#15943=AXIS2_PLACEMENT_3D('',#23591,#18566,#18567) ;
#15944=AXIS2_PLACEMENT_3D('',#23593,#18568,#18569) ;
#15945=AXIS2_PLACEMENT_3D('',#23595,#18571,#18572) ;
#15946=AXIS2_PLACEMENT_3D('',#23599,#18574,#18575) ;
#15947=AXIS2_PLACEMENT_3D('',#23600,#18576,#18577) ;
#15948=AXIS2_PLACEMENT_3D('',#23603,#18579,#18580) ;
#15949=AXIS2_PLACEMENT_3D('',#23604,#18581,#18582) ;
#15950=AXIS2_PLACEMENT_3D('',#23608,#18584,#18585) ;
#15951=AXIS2_PLACEMENT_3D('',#23609,#18586,#18587) ;
#15952=AXIS2_PLACEMENT_3D('',#23612,#18589,#18590) ;
#15953=AXIS2_PLACEMENT_3D('',#23613,#18591,#18592) ;
#15954=AXIS2_PLACEMENT_3D('',#23617,#18594,#18595) ;
#15955=AXIS2_PLACEMENT_3D('',#23618,#18596,#18597) ;
#15956=AXIS2_PLACEMENT_3D('',#23621,#18599,#18600) ;
#15957=AXIS2_PLACEMENT_3D('',#23622,#18601,#18602) ;
#15958=AXIS2_PLACEMENT_3D('',#23626,#18604,#18605) ;
#15959=AXIS2_PLACEMENT_3D('',#23627,#18606,#18607) ;
#15960=AXIS2_PLACEMENT_3D('',#23630,#18609,#18610) ;
#15961=AXIS2_PLACEMENT_3D('',#23631,#18611,#18612) ;
#15962=AXIS2_PLACEMENT_3D('',#23635,#18614,#18615) ;
#15963=AXIS2_PLACEMENT_3D('',#23636,#18616,#18617) ;
#15964=AXIS2_PLACEMENT_3D('',#23639,#18619,#18620) ;
#15965=AXIS2_PLACEMENT_3D('',#23640,#18621,#18622) ;
#15966=AXIS2_PLACEMENT_3D('',#23644,#18624,#18625) ;
#15967=AXIS2_PLACEMENT_3D('',#23645,#18626,#18627) ;
#15968=AXIS2_PLACEMENT_3D('',#23648,#18629,#18630) ;
#15969=AXIS2_PLACEMENT_3D('',#23649,#18631,#18632) ;
#15970=AXIS2_PLACEMENT_3D('',#23653,#18634,#18635) ;
#15971=AXIS2_PLACEMENT_3D('',#23654,#18636,#18637) ;
#15972=AXIS2_PLACEMENT_3D('',#23657,#18639,#18640) ;
#15973=AXIS2_PLACEMENT_3D('',#23658,#18641,#18642) ;
#15974=AXIS2_PLACEMENT_3D('',#23662,#18644,#18645) ;
#15975=AXIS2_PLACEMENT_3D('',#23663,#18646,#18647) ;
#15976=AXIS2_PLACEMENT_3D('',#23666,#18649,#18650) ;
#15977=AXIS2_PLACEMENT_3D('',#23667,#18651,#18652) ;
#15978=AXIS2_PLACEMENT_3D('',#23669,#18653,#18654) ;
#15979=AXIS2_PLACEMENT_3D('',#23672,#18656,#18657) ;
#15980=AXIS2_PLACEMENT_3D('',#23673,#18658,#18659) ;
#15981=AXIS2_PLACEMENT_3D('',#23682,#18664,#18665) ;
#15982=AXIS2_PLACEMENT_3D('',#23688,#18669,#18670) ;
#15983=AXIS2_PLACEMENT_3D('',#23694,#18674,#18675) ;
#15984=AXIS2_PLACEMENT_3D('',#23697,#18678,#18679) ;
#15985=AXIS2_PLACEMENT_3D('',#23698,#18680,#18681) ;
#18445=DIRECTION('axis',(0.,0.,1.)) ;
#18446=DIRECTION('refdir',(1.,0.,0.)) ;
#18447=DIRECTION('center_axis',(0.,0.,-1.)) ;
#18448=DIRECTION('ref_axis',(-1.,0.,0.)) ;
#18449=DIRECTION('',(0.85716730070211,-1.04972719113862E-16,-0.515038074910058)) ;
#18450=DIRECTION('center_axis',(0.,0.,1.)) ;
#18451=DIRECTION('ref_axis',(-1.,0.,0.)) ;
#18452=DIRECTION('center_axis',(0.,0.,1.)) ;
#18453=DIRECTION('ref_axis',(-1.,0.,0.)) ;
#18454=DIRECTION('center_axis',(0.,0.,1.)) ;
#18455=DIRECTION('ref_axis',(-1.,0.,0.)) ;
#18456=DIRECTION('',(0.,0.,1.)) ;
#18457=DIRECTION('center_axis',(0.,0.,-1.)) ;
#18458=DIRECTION('ref_axis',(-1.,0.,0.)) ;
#18459=DIRECTION('',(0.85716730070211,-1.04972719113862E-16,-0.515038074910058)) ;
#18460=DIRECTION('center_axis',(0.,0.,1.)) ;
#18461=DIRECTION('ref_axis',(-1.,0.,0.)) ;
#18462=DIRECTION('center_axis',(0.,0.,1.)) ;
#18463=DIRECTION('ref_axis',(-1.,0.,0.)) ;
#18464=DIRECTION('center_axis',(0.,0.,1.)) ;
#18465=DIRECTION('ref_axis',(-1.,0.,0.)) ;
#18466=DIRECTION('',(0.,0.,1.)) ;
#18467=DIRECTION('center_axis',(-9.473903143468E-16,1.,0.)) ;
#18468=DIRECTION('ref_axis',(0.,0.,1.)) ;
#18469=DIRECTION('',(-5.92914802803472E-16,0.515038074910058,-0.85716730070211)) ;
#18470=DIRECTION('center_axis',(9.473903143468E-16,-1.,0.)) ;
#18471=DIRECTION('ref_axis',(0.,0.,1.)) ;
#18472=DIRECTION('center_axis',(9.473903143468E-16,-1.,0.)) ;
#18473=DIRECTION('ref_axis',(0.,0.,1.)) ;
#18474=DIRECTION('center_axis',(9.47390314346801E-16,-1.,0.)) ;
#18475=DIRECTION('ref_axis',(0.,0.,1.)) ;
#18476=DIRECTION('',(9.473903143468E-16,-1.,0.)) ;
#18477=DIRECTION('center_axis',(-9.473903143468E-16,1.,0.)) ;
#18478=DIRECTION('ref_axis',(0.,0.,1.)) ;
#18479=DIRECTION('',(-5.92914802803472E-16,0.515038074910058,-0.85716730070211)) ;
#18480=DIRECTION('center_axis',(9.473903143468E-16,-1.,0.)) ;
#18481=DIRECTION('ref_axis',(0.,0.,1.)) ;
#18482=DIRECTION('center_axis',(9.473903143468E-16,-1.,0.)) ;
#18483=DIRECTION('ref_axis',(0.,0.,1.)) ;
#18484=DIRECTION('center_axis',(9.47390314346801E-16,-1.,0.)) ;
#18485=DIRECTION('ref_axis',(0.,0.,1.)) ;
#18486=DIRECTION('',(9.473903143468E-16,-1.,0.)) ;
#18487=DIRECTION('center_axis',(-3.5527136788005E-16,-1.,0.)) ;
#18488=DIRECTION('ref_axis',(0.,0.,-1.)) ;
#18489=DIRECTION('',(-2.87951000497466E-16,-0.515038074910058,0.85716730070211)) ;
#18490=DIRECTION('center_axis',(3.5527136788005E-16,1.,0.)) ;
#18491=DIRECTION('ref_axis',(0.,0.,-1.)) ;
#18492=DIRECTION('center_axis',(3.5527136788005E-16,1.,0.)) ;
#18493=DIRECTION('ref_axis',(0.,0.,-1.)) ;
#18494=DIRECTION('center_axis',(4.2632564145606E-15,1.,0.)) ;
#18495=DIRECTION('ref_axis',(0.,0.,-1.)) ;
#18496=DIRECTION('',(3.5527136788005E-16,1.,0.)) ;
#18497=DIRECTION('center_axis',(-3.5527136788005E-16,-1.,0.)) ;
#18498=DIRECTION('ref_axis',(0.,0.,-1.)) ;
#18499=DIRECTION('',(-2.87951000497466E-16,-0.515038074910058,0.85716730070211)) ;
#18500=DIRECTION('center_axis',(3.5527136788005E-16,1.,0.)) ;
#18501=DIRECTION('ref_axis',(0.,0.,-1.)) ;
#18502=DIRECTION('center_axis',(3.5527136788005E-16,1.,0.)) ;
#18503=DIRECTION('ref_axis',(0.,0.,-1.)) ;
#18504=DIRECTION('center_axis',(4.2632564145606E-15,1.,0.)) ;
#18505=DIRECTION('ref_axis',(0.,0.,-1.)) ;
#18506=DIRECTION('',(3.5527136788005E-16,1.,0.)) ;
#18507=DIRECTION('center_axis',(0.,0.,-1.)) ;
#18508=DIRECTION('ref_axis',(1.,0.,0.)) ;
#18509=DIRECTION('center_axis',(0.,0.,-1.)) ;
#18510=DIRECTION('ref_axis',(1.,0.,0.)) ;
#18511=DIRECTION('center_axis',(0.,0.,-1.)) ;
#18512=DIRECTION('ref_axis',(1.,0.,0.)) ;
#18513=DIRECTION('center_axis',(0.,0.,-1.)) ;
#18514=DIRECTION('ref_axis',(1.,0.,0.)) ;
#18515=DIRECTION('',(0.,0.,-1.)) ;
#18516=DIRECTION('center_axis',(0.,0.,-1.)) ;
#18517=DIRECTION('ref_axis',(1.,0.,0.)) ;
#18518=DIRECTION('center_axis',(0.,0.,-1.)) ;
#18519=DIRECTION('ref_axis',(1.,0.,0.)) ;
#18520=DIRECTION('center_axis',(0.,0.,1.)) ;
#18521=DIRECTION('ref_axis',(1.,0.,0.)) ;
#18522=DIRECTION('',(0.,0.,-1.)) ;
#18523=DIRECTION('center_axis',(0.,0.,-1.)) ;
#18524=DIRECTION('ref_axis',(1.,0.,0.)) ;
#18525=DIRECTION('center_axis',(0.,0.,-1.)) ;
#18526=DIRECTION('ref_axis',(1.,0.,0.)) ;
#18527=DIRECTION('center_axis',(0.,0.,-1.)) ;
#18528=DIRECTION('ref_axis',(1.,0.,0.)) ;
#18529=DIRECTION('center_axis',(0.,0.,-1.)) ;
#18530=DIRECTION('ref_axis',(1.,0.,0.)) ;
#18531=DIRECTION('',(0.,0.,-1.)) ;
#18532=DIRECTION('center_axis',(0.,0.,-1.)) ;
#18533=DIRECTION('ref_axis',(1.,0.,0.)) ;
#18534=DIRECTION('center_axis',(0.,0.,-1.)) ;
#18535=DIRECTION('ref_axis',(1.,0.,0.)) ;
#18536=DIRECTION('center_axis',(0.,0.,1.)) ;
#18537=DIRECTION('ref_axis',(1.,0.,0.)) ;
#18538=DIRECTION('',(0.,0.,-1.)) ;
#18539=DIRECTION('center_axis',(0.,0.,-1.)) ;
#18540=DIRECTION('ref_axis',(1.,0.,0.)) ;
#18541=DIRECTION('center_axis',(0.,0.,-1.)) ;
#18542=DIRECTION('ref_axis',(1.,0.,0.)) ;
#18543=DIRECTION('center_axis',(0.,0.,-1.)) ;
#18544=DIRECTION('ref_axis',(1.,0.,0.)) ;
#18545=DIRECTION('center_axis',(0.,0.,-1.)) ;
#18546=DIRECTION('ref_axis',(1.,0.,0.)) ;
#18547=DIRECTION('',(0.,0.,-1.)) ;
#18548=DIRECTION('center_axis',(0.,0.,-1.)) ;
#18549=DIRECTION('ref_axis',(1.,0.,0.)) ;
#18550=DIRECTION('center_axis',(0.,0.,-1.)) ;
#18551=DIRECTION('ref_axis',(1.,0.,0.)) ;
#18552=DIRECTION('center_axis',(0.,0.,1.)) ;
#18553=DIRECTION('ref_axis',(1.,0.,0.)) ;
#18554=DIRECTION('',(0.,0.,-1.)) ;
#18555=DIRECTION('center_axis',(0.,0.,-1.)) ;
#18556=DIRECTION('ref_axis',(1.,0.,0.)) ;
#18557=DIRECTION('center_axis',(0.,0.,-1.)) ;
#18558=DIRECTION('ref_axis',(1.,0.,0.)) ;
#18559=DIRECTION('center_axis',(0.,0.,-1.)) ;
#18560=DIRECTION('ref_axis',(1.,0.,0.)) ;
#18561=DIRECTION('center_axis',(0.,0.,-1.)) ;
#18562=DIRECTION('ref_axis',(1.,0.,0.)) ;
#18563=DIRECTION('',(0.,0.,-1.)) ;
#18564=DIRECTION('center_axis',(0.,0.,-1.)) ;
#18565=DIRECTION('ref_axis',(1.,0.,0.)) ;
#18566=DIRECTION('center_axis',(0.,0.,-1.)) ;
#18567=DIRECTION('ref_axis',(1.,0.,0.)) ;
#18568=DIRECTION('center_axis',(0.,0.,1.)) ;
#18569=DIRECTION('ref_axis',(1.,0.,0.)) ;
#18570=DIRECTION('',(0.,0.,-1.)) ;
#18571=DIRECTION('center_axis',(0.,0.,1.)) ;
#18572=DIRECTION('ref_axis',(-1.,0.,0.)) ;
#18573=DIRECTION('',(0.85716730070211,1.04972719113862E-16,0.515038074910058)) ;
#18574=DIRECTION('center_axis',(0.,0.,1.)) ;
#18575=DIRECTION('ref_axis',(-1.,0.,0.)) ;
#18576=DIRECTION('center_axis',(0.,0.,1.)) ;
#18577=DIRECTION('ref_axis',(-1.,0.,0.)) ;
#18578=DIRECTION('',(0.,0.,1.)) ;
#18579=DIRECTION('center_axis',(0.,0.,1.)) ;
#18580=DIRECTION('ref_axis',(-1.,0.,0.)) ;
#18581=DIRECTION('center_axis',(0.,0.,1.)) ;
#18582=DIRECTION('ref_axis',(-1.,0.,0.)) ;
#18583=DIRECTION('',(0.85716730070211,1.04972719113862E-16,0.515038074910058)) ;
#18584=DIRECTION('center_axis',(0.,0.,1.)) ;
#18585=DIRECTION('ref_axis',(-1.,0.,0.)) ;
#18586=DIRECTION('center_axis',(0.,0.,1.)) ;
#18587=DIRECTION('ref_axis',(-1.,0.,0.)) ;
#18588=DIRECTION('',(0.,0.,1.)) ;
#18589=DIRECTION('center_axis',(0.,0.,-1.)) ;
#18590=DIRECTION('ref_axis',(-1.,0.,0.)) ;
#18591=DIRECTION('center_axis',(0.,0.,1.)) ;
#18592=DIRECTION('ref_axis',(-1.,0.,0.)) ;
#18593=DIRECTION('',(0.85716730070211,1.04972719113862E-16,0.515038074910058)) ;
#18594=DIRECTION('center_axis',(0.,0.,1.)) ;
#18595=DIRECTION('ref_axis',(-1.,0.,0.)) ;
#18596=DIRECTION('center_axis',(0.,0.,1.)) ;
#18597=DIRECTION('ref_axis',(-1.,0.,0.)) ;
#18598=DIRECTION('',(0.,0.,1.)) ;
#18599=DIRECTION('center_axis',(0.,0.,-1.)) ;
#18600=DIRECTION('ref_axis',(-1.,0.,0.)) ;
#18601=DIRECTION('center_axis',(0.,0.,1.)) ;
#18602=DIRECTION('ref_axis',(-1.,0.,0.)) ;
#18603=DIRECTION('',(0.85716730070211,1.04972719113862E-16,0.515038074910058)) ;
#18604=DIRECTION('center_axis',(0.,0.,1.)) ;
#18605=DIRECTION('ref_axis',(-1.,0.,0.)) ;
#18606=DIRECTION('center_axis',(0.,0.,1.)) ;
#18607=DIRECTION('ref_axis',(-1.,0.,0.)) ;
#18608=DIRECTION('',(0.,0.,1.)) ;
#18609=DIRECTION('center_axis',(0.,0.,-1.)) ;
#18610=DIRECTION('ref_axis',(-1.,0.,0.)) ;
#18611=DIRECTION('center_axis',(0.,0.,1.)) ;
#18612=DIRECTION('ref_axis',(-1.,0.,0.)) ;
#18613=DIRECTION('',(0.85716730070211,1.04972719113862E-16,0.515038074910058)) ;
#18614=DIRECTION('center_axis',(0.,0.,1.)) ;
#18615=DIRECTION('ref_axis',(-1.,0.,0.)) ;
#18616=DIRECTION('center_axis',(0.,0.,1.)) ;
#18617=DIRECTION('ref_axis',(-1.,0.,0.)) ;
#18618=DIRECTION('',(0.,0.,1.)) ;
#18619=DIRECTION('center_axis',(0.,0.,-1.)) ;
#18620=DIRECTION('ref_axis',(-1.,0.,0.)) ;
#18621=DIRECTION('center_axis',(0.,0.,1.)) ;
#18622=DIRECTION('ref_axis',(-1.,0.,0.)) ;
#18623=DIRECTION('',(0.85716730070211,1.04972719113862E-16,0.515038074910058)) ;
#18624=DIRECTION('center_axis',(0.,0.,1.)) ;
#18625=DIRECTION('ref_axis',(-1.,0.,0.)) ;
#18626=DIRECTION('center_axis',(0.,0.,1.)) ;
#18627=DIRECTION('ref_axis',(-1.,0.,0.)) ;
#18628=DIRECTION('',(0.,0.,1.)) ;
#18629=DIRECTION('center_axis',(0.,0.,-1.)) ;
#18630=DIRECTION('ref_axis',(-1.,0.,0.)) ;
#18631=DIRECTION('center_axis',(0.,0.,1.)) ;
#18632=DIRECTION('ref_axis',(-1.,0.,0.)) ;
#18633=DIRECTION('',(0.85716730070211,1.04972719113862E-16,0.515038074910058)) ;
#18634=DIRECTION('center_axis',(0.,0.,1.)) ;
#18635=DIRECTION('ref_axis',(-1.,0.,0.)) ;
#18636=DIRECTION('center_axis',(0.,0.,1.)) ;
#18637=DIRECTION('ref_axis',(-1.,0.,0.)) ;
#18638=DIRECTION('',(0.,0.,1.)) ;
#18639=DIRECTION('center_axis',(0.,0.,-1.)) ;
#18640=DIRECTION('ref_axis',(-1.,0.,0.)) ;
#18641=DIRECTION('center_axis',(0.,0.,1.)) ;
#18642=DIRECTION('ref_axis',(-1.,0.,0.)) ;
#18643=DIRECTION('',(0.85716730070211,1.04972719113862E-16,0.515038074910058)) ;
#18644=DIRECTION('center_axis',(0.,0.,1.)) ;
#18645=DIRECTION('ref_axis',(-1.,0.,0.)) ;
#18646=DIRECTION('center_axis',(0.,0.,1.)) ;
#18647=DIRECTION('ref_axis',(-1.,0.,0.)) ;
#18648=DIRECTION('',(0.,0.,1.)) ;
#18649=DIRECTION('center_axis',(0.,0.,1.)) ;
#18650=DIRECTION('ref_axis',(-1.,0.,0.)) ;
#18651=DIRECTION('center_axis',(0.,0.,-1.)) ;
#18652=DIRECTION('ref_axis',(1.,0.,0.)) ;
#18653=DIRECTION('center_axis',(0.,0.,1.)) ;
#18654=DIRECTION('ref_axis',(1.,0.,0.)) ;
#18655=DIRECTION('',(0.,0.,-1.)) ;
#18656=DIRECTION('center_axis',(0.,0.,-1.)) ;
#18657=DIRECTION('ref_axis',(1.,0.,0.)) ;
#18658=DIRECTION('center_axis',(4.2632564145606E-15,1.,0.)) ;
#18659=DIRECTION('ref_axis',(-1.,4.2632564145606E-15,0.)) ;
#18660=DIRECTION('',(1.,-4.2632564145606E-15,0.)) ;
#18661=DIRECTION('',(0.,0.,1.)) ;
#18662=DIRECTION('',(-1.,4.2632564145606E-15,0.)) ;
#18663=DIRECTION('',(0.,0.,1.)) ;
#18664=DIRECTION('center_axis',(-1.,2.66453525910036E-16,0.)) ;
#18665=DIRECTION('ref_axis',(-2.66453525910036E-16,-1.,0.)) ;
#18666=DIRECTION('',(2.66453525910036E-16,1.,0.)) ;
#18667=DIRECTION('',(0.,0.,1.)) ;
#18668=DIRECTION('',(-2.66453525910036E-16,-1.,0.)) ;
#18669=DIRECTION('center_axis',(9.47390314346801E-16,-1.,0.)) ;
#18670=DIRECTION('ref_axis',(1.,9.47390314346801E-16,0.)) ;
#18671=DIRECTION('',(1.,9.47390314346801E-16,0.)) ;
#18672=DIRECTION('',(0.,0.,1.)) ;
#18673=DIRECTION('',(1.,9.47390314346801E-16,0.)) ;
#18674=DIRECTION('center_axis',(1.,-1.68753899743024E-15,0.)) ;
#18675=DIRECTION('ref_axis',(1.68753899743024E-15,1.,0.)) ;
#18676=DIRECTION('',(-1.68753899743024E-15,-1.,0.)) ;
#18677=DIRECTION('',(1.68753899743024E-15,1.,0.)) ;
#18678=DIRECTION('center_axis',(0.,0.,1.)) ;
#18679=DIRECTION('ref_axis',(1.,0.,0.)) ;
#18680=DIRECTION('center_axis',(0.,0.,1.)) ;
#18681=DIRECTION('ref_axis',(1.,0.,0.)) ;
#23488=CARTESIAN_POINT('',(0.,0.,0.)) ;
#23489=CARTESIAN_POINT('Origin',(63.,219.45,9.78673043802305)) ;
#23490=CARTESIAN_POINT('',(63.,219.45,10.5120219304813)) ;
#23491=CARTESIAN_POINT('',(65.117,219.45,9.24)) ;
#23492=CARTESIAN_POINT('',(64.2070877496217,219.45,9.78673043802305)) ;
#23493=CARTESIAN_POINT('Origin',(63.,219.45,9.24)) ;
#23494=CARTESIAN_POINT('Origin',(63.,219.45,4.23999999999999)) ;
#23495=CARTESIAN_POINT('',(65.117,219.45,0.)) ;
#23496=CARTESIAN_POINT('Origin',(63.,219.45,0.)) ;
#23497=CARTESIAN_POINT('',(65.117,219.45,4.23999999999999)) ;
#23498=CARTESIAN_POINT('Origin',(-62.9999999999999,219.45,9.78673043802305)) ;
#23499=CARTESIAN_POINT('',(-62.9999999999999,219.45,10.5120219304813)) ;
#23500=CARTESIAN_POINT('',(-60.8829999999999,219.45,9.24)) ;
#23501=CARTESIAN_POINT('',(-61.7929122503782,219.45,9.78673043802305)) ;
#23502=CARTESIAN_POINT('Origin',(-62.9999999999999,219.45,9.24)) ;
#23503=CARTESIAN_POINT('Origin',(-62.9999999999999,219.45,4.23999999999999)) ;
#23504=CARTESIAN_POINT('',(-60.8829999999999,219.45,0.)) ;
#23505=CARTESIAN_POINT('Origin',(-62.9999999999999,219.45,0.)) ;
#23506=CARTESIAN_POINT('',(-60.8829999999999,219.45,4.23999999999999)) ;
#23507=CARTESIAN_POINT('Origin',(44.9999999999989,385.343736383858,12.)) ;
#23508=CARTESIAN_POINT('',(44.9999999999989,383.888531181086,12.)) ;
#23509=CARTESIAN_POINT('',(44.9999999999989,386.45,7.73699999999999)) ;
#23510=CARTESIAN_POINT('',(44.9999999999989,385.343736383858,9.57813183841693)) ;
#23511=CARTESIAN_POINT('Origin',(44.9999999999989,386.45,12.)) ;
#23512=CARTESIAN_POINT('Origin',(44.9999999999989,405.45,12.)) ;
#23513=CARTESIAN_POINT('',(44.9999999999989,409.45,7.73699999999999)) ;
#23514=CARTESIAN_POINT('Origin',(44.9999999999989,409.45,12.)) ;
#23515=CARTESIAN_POINT('',(44.9999999999989,405.45,7.737)) ;
#23516=CARTESIAN_POINT('Origin',(-45.0000000000005,385.343736383858,12.)) ;
#23517=CARTESIAN_POINT('',(-45.0000000000005,383.888531181086,12.)) ;
#23518=CARTESIAN_POINT('',(-45.0000000000005,386.45,7.73699999999999)) ;
#23519=CARTESIAN_POINT('',(-45.0000000000005,385.343736383858,9.57813183841693)) ;
#23520=CARTESIAN_POINT('Origin',(-45.0000000000005,386.45,12.)) ;
#23521=CARTESIAN_POINT('Origin',(-45.0000000000005,405.45,12.)) ;
#23522=CARTESIAN_POINT('',(-45.0000000000005,409.45,7.73699999999999)) ;
#23523=CARTESIAN_POINT('Origin',(-45.0000000000005,409.45,12.)) ;
#23524=CARTESIAN_POINT('',(-45.0000000000005,405.45,7.737)) ;
#23525=CARTESIAN_POINT('Origin',(44.9999999999995,228.556263616143,12.)) ;
#23526=CARTESIAN_POINT('',(44.9999999999995,230.011468818915,12.)) ;
#23527=CARTESIAN_POINT('',(44.9999999999995,227.45,16.263)) ;
#23528=CARTESIAN_POINT('',(44.9999999999995,228.556263616143,14.4218681615831)) ;
#23529=CARTESIAN_POINT('Origin',(44.9999999999995,227.45,12.)) ;
#23530=CARTESIAN_POINT('Origin',(44.9999999999995,208.45,12.)) ;
#23531=CARTESIAN_POINT('',(44.9999999999995,209.449999999999,16.263)) ;
#23532=CARTESIAN_POINT('Origin',(44.9999999999995,209.449999999999,12.)) ;
#23533=CARTESIAN_POINT('',(44.9999999999995,208.45,16.263)) ;
#23534=CARTESIAN_POINT('Origin',(-44.9999999999999,228.556263616143,12.)) ;
#23535=CARTESIAN_POINT('',(-44.9999999999999,230.011468818915,12.)) ;
#23536=CARTESIAN_POINT('',(-44.9999999999999,227.45,16.263)) ;
#23537=CARTESIAN_POINT('',(-44.9999999999999,228.556263616143,14.4218681615831)) ;
#23538=CARTESIAN_POINT('Origin',(-44.9999999999999,227.45,12.)) ;
#23539=CARTESIAN_POINT('Origin',(-44.9999999999999,208.45,12.)) ;
#23540=CARTESIAN_POINT('',(-44.9999999999999,209.449999999999,16.263)) ;
#23541=CARTESIAN_POINT('Origin',(-44.9999999999999,209.449999999999,12.)) ;
#23542=CARTESIAN_POINT('',(-44.9999999999999,208.45,16.263)) ;
#23543=CARTESIAN_POINT('Origin',(-62.9999999999999,239.45,10.)) ;
#23544=CARTESIAN_POINT('',(-71.9999999999999,239.45,10.)) ;
#23545=CARTESIAN_POINT('Origin',(-62.9999999999999,239.45,10.)) ;
#23546=CARTESIAN_POINT('',(-68.4999999999999,239.45,10.)) ;
#23547=CARTESIAN_POINT('Origin',(-62.9999999999999,239.45,10.)) ;
#23548=CARTESIAN_POINT('Origin',(-62.9999999999999,239.45,5.)) ;
#23549=CARTESIAN_POINT('',(-71.9999999999999,239.45,0.)) ;
#23550=CARTESIAN_POINT('',(-71.9999999999999,239.45,5.)) ;
#23551=CARTESIAN_POINT('Origin',(-62.9999999999999,239.45,0.)) ;
#23552=CARTESIAN_POINT('Origin',(-62.9999999999999,239.45,19.)) ;
#23553=CARTESIAN_POINT('',(-68.4999999999999,239.45,24.)) ;
#23554=CARTESIAN_POINT('Origin',(-62.9999999999999,239.45,24.)) ;
#23555=CARTESIAN_POINT('',(-68.4999999999999,239.45,19.)) ;
#23556=CARTESIAN_POINT('Origin',(63.,379.45,10.)) ;
#23557=CARTESIAN_POINT('',(54.,379.45,10.)) ;
#23558=CARTESIAN_POINT('Origin',(63.,379.45,10.)) ;
#23559=CARTESIAN_POINT('',(57.5,379.45,10.)) ;
#23560=CARTESIAN_POINT('Origin',(63.,379.45,10.)) ;
#23561=CARTESIAN_POINT('Origin',(63.,379.45,5.)) ;
#23562=CARTESIAN_POINT('',(54.,379.45,0.)) ;
#23563=CARTESIAN_POINT('',(54.,379.45,5.)) ;
#23564=CARTESIAN_POINT('Origin',(63.,379.45,0.)) ;
#23565=CARTESIAN_POINT('Origin',(63.,379.45,19.)) ;
#23566=CARTESIAN_POINT('',(57.5,379.45,24.)) ;
#23567=CARTESIAN_POINT('Origin',(63.,379.45,24.)) ;
#23568=CARTESIAN_POINT('',(57.5,379.45,19.)) ;
#23569=CARTESIAN_POINT('Origin',(63.,239.45,10.)) ;
#23570=CARTESIAN_POINT('',(54.,239.45,10.)) ;
#23571=CARTESIAN_POINT('Origin',(63.,239.45,10.)) ;
#23572=CARTESIAN_POINT('',(57.5,239.45,10.)) ;
#23573=CARTESIAN_POINT('Origin',(63.,239.45,10.)) ;
#23574=CARTESIAN_POINT('Origin',(63.,239.45,5.)) ;
#23575=CARTESIAN_POINT('',(54.,239.45,0.)) ;
#23576=CARTESIAN_POINT('',(54.,239.45,5.)) ;
#23577=CARTESIAN_POINT('Origin',(63.,239.45,0.)) ;
#23578=CARTESIAN_POINT('Origin',(63.,239.45,19.)) ;
#23579=CARTESIAN_POINT('',(57.5,239.45,24.)) ;
#23580=CARTESIAN_POINT('Origin',(63.,239.45,24.)) ;
#23581=CARTESIAN_POINT('',(57.5,239.45,19.)) ;
#23582=CARTESIAN_POINT('Origin',(-62.9999999999999,379.45,10.)) ;
#23583=CARTESIAN_POINT('',(-71.9999999999999,379.45,10.)) ;
#23584=CARTESIAN_POINT('Origin',(-62.9999999999999,379.45,10.)) ;
#23585=CARTESIAN_POINT('',(-68.4999999999999,379.45,10.)) ;
#23586=CARTESIAN_POINT('Origin',(-62.9999999999999,379.45,10.)) ;
#23587=CARTESIAN_POINT('Origin',(-62.9999999999999,379.45,5.)) ;
#23588=CARTESIAN_POINT('',(-71.9999999999999,379.45,0.)) ;
#23589=CARTESIAN_POINT('',(-71.9999999999999,379.45,5.)) ;
#23590=CARTESIAN_POINT('Origin',(-62.9999999999999,379.45,0.)) ;
#23591=CARTESIAN_POINT('Origin',(-62.9999999999999,379.45,19.)) ;
#23592=CARTESIAN_POINT('',(-68.4999999999999,379.45,24.)) ;
#23593=CARTESIAN_POINT('Origin',(-62.9999999999999,379.45,24.)) ;
#23594=CARTESIAN_POINT('',(-68.4999999999999,379.45,19.)) ;
#23595=CARTESIAN_POINT('Origin',(45.,354.45,13.0085799786045)) ;
#23596=CARTESIAN_POINT('',(45.,354.45,12.0171599572091)) ;
#23597=CARTESIAN_POINT('',(48.3,354.45,14.)) ;
#23598=CARTESIAN_POINT('',(46.65,354.45,13.0085799786045)) ;
#23599=CARTESIAN_POINT('Origin',(45.,354.45,14.)) ;
#23600=CARTESIAN_POINT('Origin',(45.,354.45,22.)) ;
#23601=CARTESIAN_POINT('',(48.3,354.45,24.)) ;
#23602=CARTESIAN_POINT('',(48.3,354.45,22.)) ;
#23603=CARTESIAN_POINT('Origin',(45.,354.45,24.)) ;
#23604=CARTESIAN_POINT('Origin',(-5.51091059616309E-15,399.45,13.3540332243106)) ;
#23605=CARTESIAN_POINT('',(-5.67105257905314E-15,399.45,12.4873333915981)) ;
#23606=CARTESIAN_POINT('',(2.51749999999999,399.45,14.)) ;
#23607=CARTESIAN_POINT('',(1.44243074893997,399.45,13.3540332243106)) ;
#23608=CARTESIAN_POINT('Origin',(-5.51091059616309E-15,399.45,14.)) ;
#23609=CARTESIAN_POINT('Origin',(-5.51091059616309E-15,399.45,22.)) ;
#23610=CARTESIAN_POINT('',(2.51749999999999,399.45,24.)) ;
#23611=CARTESIAN_POINT('',(2.51749999999999,399.45,22.)) ;
#23612=CARTESIAN_POINT('Origin',(-5.51091059616309E-15,399.45,24.)) ;
#23613=CARTESIAN_POINT('Origin',(-45.,354.45,13.3540332243106)) ;
#23614=CARTESIAN_POINT('',(-45.,354.45,12.4873333915981)) ;
#23615=CARTESIAN_POINT('',(-42.4825,354.45,14.)) ;
#23616=CARTESIAN_POINT('',(-43.55756925106,354.45,13.3540332243106)) ;
#23617=CARTESIAN_POINT('Origin',(-45.,354.45,14.)) ;
#23618=CARTESIAN_POINT('Origin',(-45.,354.45,22.)) ;
#23619=CARTESIAN_POINT('',(-42.4825,354.45,24.)) ;
#23620=CARTESIAN_POINT('',(-42.4825,354.45,22.)) ;
#23621=CARTESIAN_POINT('Origin',(-45.,354.45,24.)) ;
#23622=CARTESIAN_POINT('Origin',(0.,309.45,13.3540332243106)) ;
#23623=CARTESIAN_POINT('',(-1.60141982890047E-16,309.45,12.4873333915981)) ;
#23624=CARTESIAN_POINT('',(2.5175,309.45,14.)) ;
#23625=CARTESIAN_POINT('',(1.44243074893998,309.45,13.3540332243106)) ;
#23626=CARTESIAN_POINT('Origin',(0.,309.45,14.)) ;
#23627=CARTESIAN_POINT('Origin',(0.,309.45,22.)) ;
#23628=CARTESIAN_POINT('',(2.5175,309.45,24.)) ;
#23629=CARTESIAN_POINT('',(2.5175,309.45,22.)) ;
#23630=CARTESIAN_POINT('Origin',(0.,309.45,24.)) ;
#23631=CARTESIAN_POINT('Origin',(-31.8198051533946,322.630194846605,13.3540332243106)) ;
#23632=CARTESIAN_POINT('',(-31.8198051533946,322.630194846605,12.4873333915981)) ;
#23633=CARTESIAN_POINT('',(-29.3023051533946,322.630194846605,14.)) ;
#23634=CARTESIAN_POINT('',(-30.3773744044546,322.630194846605,13.3540332243106)) ;
#23635=CARTESIAN_POINT('Origin',(-31.8198051533946,322.630194846605,14.)) ;
#23636=CARTESIAN_POINT('Origin',(-31.8198051533946,322.630194846605,22.)) ;
#23637=CARTESIAN_POINT('',(-29.3023051533946,322.630194846605,24.)) ;
#23638=CARTESIAN_POINT('',(-29.3023051533946,322.630194846605,22.)) ;
#23639=CARTESIAN_POINT('Origin',(-31.8198051533946,322.630194846605,24.)) ;
#23640=CARTESIAN_POINT('Origin',(-31.8198051533946,386.269805153395,13.3540332243106)) ;
#23641=CARTESIAN_POINT('',(-31.8198051533946,386.269805153395,12.4873333915981)) ;
#23642=CARTESIAN_POINT('',(-29.3023051533946,386.269805153395,14.)) ;
#23643=CARTESIAN_POINT('',(-30.3773744044546,386.269805153395,13.3540332243106)) ;
#23644=CARTESIAN_POINT('Origin',(-31.8198051533946,386.269805153395,14.)) ;
#23645=CARTESIAN_POINT('Origin',(-31.8198051533946,386.269805153395,22.)) ;
#23646=CARTESIAN_POINT('',(-29.3023051533946,386.269805153395,24.)) ;
#23647=CARTESIAN_POINT('',(-29.3023051533946,386.269805153395,22.)) ;
#23648=CARTESIAN_POINT('Origin',(-31.8198051533946,386.269805153395,24.)) ;
#23649=CARTESIAN_POINT('Origin',(31.8198051533946,386.269805153395,13.3540332243106)) ;
#23650=CARTESIAN_POINT('',(31.8198051533946,386.269805153395,12.4873333915981)) ;
#23651=CARTESIAN_POINT('',(34.3373051533946,386.269805153395,14.)) ;
#23652=CARTESIAN_POINT('',(33.2622359023346,386.269805153395,13.3540332243106)) ;
#23653=CARTESIAN_POINT('Origin',(31.8198051533946,386.269805153395,14.)) ;
#23654=CARTESIAN_POINT('Origin',(31.8198051533946,386.269805153395,22.)) ;
#23655=CARTESIAN_POINT('',(34.3373051533946,386.269805153395,24.)) ;
#23656=CARTESIAN_POINT('',(34.3373051533946,386.269805153395,22.)) ;
#23657=CARTESIAN_POINT('Origin',(31.8198051533946,386.269805153395,24.)) ;
#23658=CARTESIAN_POINT('Origin',(31.8198051533946,322.630194846605,13.0085799786045)) ;
#23659=CARTESIAN_POINT('',(31.8198051533946,322.630194846605,12.0171599572091)) ;
#23660=CARTESIAN_POINT('',(35.1198051533946,322.630194846605,14.)) ;
#23661=CARTESIAN_POINT('',(33.4698051533946,322.630194846605,13.0085799786045)) ;
#23662=CARTESIAN_POINT('Origin',(31.8198051533946,322.630194846605,14.)) ;
#23663=CARTESIAN_POINT('Origin',(31.8198051533946,322.630194846605,22.)) ;
#23664=CARTESIAN_POINT('',(35.1198051533946,322.630194846605,24.)) ;
#23665=CARTESIAN_POINT('',(35.1198051533946,322.630194846605,22.)) ;
#23666=CARTESIAN_POINT('Origin',(31.8198051533946,322.630194846605,24.)) ;
#23667=CARTESIAN_POINT('Origin',(0.,354.45,0.)) ;
#23668=CARTESIAN_POINT('',(-37.5,354.45,24.)) ;
#23669=CARTESIAN_POINT('Origin',(0.,354.45,24.)) ;
#23670=CARTESIAN_POINT('',(-37.5,354.45,0.)) ;
#23671=CARTESIAN_POINT('',(-37.5,354.45,0.)) ;
#23672=CARTESIAN_POINT('Origin',(0.,354.45,0.)) ;
#23673=CARTESIAN_POINT('Origin',(75.,209.449999999999,0.)) ;
#23674=CARTESIAN_POINT('',(-75.0000000000002,209.45,0.)) ;
#23675=CARTESIAN_POINT('',(75.,209.449999999999,0.)) ;
#23676=CARTESIAN_POINT('',(-100.,209.45,0.)) ;
#23677=CARTESIAN_POINT('',(75.,209.449999999999,24.)) ;
#23678=CARTESIAN_POINT('',(75.,209.449999999999,0.)) ;
#23679=CARTESIAN_POINT('',(-75.0000000000002,209.45,24.)) ;
#23680=CARTESIAN_POINT('',(-100.,209.45,24.)) ;
#23681=CARTESIAN_POINT('',(-75.0000000000002,209.45,0.)) ;
#23682=CARTESIAN_POINT('Origin',(75.0000000000001,409.45,0.)) ;
#23683=CARTESIAN_POINT('',(75.0000000000001,409.45,0.)) ;
#23684=CARTESIAN_POINT('',(75.,209.449999999999,0.)) ;
#23685=CARTESIAN_POINT('',(75.0000000000001,409.45,24.)) ;
#23686=CARTESIAN_POINT('',(75.0000000000001,409.45,0.)) ;
#23687=CARTESIAN_POINT('',(75.,209.449999999999,24.)) ;
#23688=CARTESIAN_POINT('Origin',(-74.9999999999999,409.45,0.)) ;
#23689=CARTESIAN_POINT('',(-74.9999999999999,409.45,0.)) ;
#23690=CARTESIAN_POINT('',(-74.9999999999999,409.45,0.)) ;
#23691=CARTESIAN_POINT('',(-74.9999999999999,409.45,24.)) ;
#23692=CARTESIAN_POINT('',(-74.9999999999999,409.45,0.)) ;
#23693=CARTESIAN_POINT('',(-74.9999999999999,409.45,24.)) ;
#23694=CARTESIAN_POINT('Origin',(-75.0000000000002,209.45,0.)) ;
#23695=CARTESIAN_POINT('',(-74.9999999999999,409.45,0.)) ;
#23696=CARTESIAN_POINT('',(-74.9999999999999,409.45,24.)) ;
#23697=CARTESIAN_POINT('Origin',(-6.21724893790088E-14,309.45,0.)) ;
#23698=CARTESIAN_POINT('Origin',(-6.21724893790088E-14,309.45,24.)) ;
#63795=UNCERTAINTY_MEASURE_WITH_UNIT(LENGTH_MEASURE(0.01),#63825,
'DISTANCE_ACCURACY_VALUE',
'Maximum model space distance between geometric entities at asserted c
onnectivities') ;
#63807=UNCERTAINTY_MEASURE_WITH_UNIT(LENGTH_MEASURE(0.01),#63825,
'DISTANCE_ACCURACY_VALUE',
'Maximum model space distance between geometric entities at asserted c
onnectivities') ;
#63812=(
GEOMETRIC_REPRESENTATION_CONTEXT(3)
GLOBAL_UNCERTAINTY_ASSIGNED_CONTEXT((#63795))
GLOBAL_UNIT_ASSIGNED_CONTEXT((#63825,#63827,#63828))
REPRESENTATION_CONTEXT('','3D')
) ;
#63824=(
GEOMETRIC_REPRESENTATION_CONTEXT(3)
GLOBAL_UNCERTAINTY_ASSIGNED_CONTEXT((#63807))
GLOBAL_UNIT_ASSIGNED_CONTEXT((#63825,#63827,#63828))
REPRESENTATION_CONTEXT('','3D')
) ;
#63825=(
LENGTH_UNIT()
NAMED_UNIT(*)
SI_UNIT(.MILLI.,.METRE.)
) ;
#63827=(
NAMED_UNIT(*)
PLANE_ANGLE_UNIT()
SI_UNIT($,.RADIAN.)
) ;
#63828=(
NAMED_UNIT(*)
SI_UNIT($,.STERADIAN.)
SOLID_ANGLE_UNIT()
) ;
#63833=SHAPE_DEFINITION_REPRESENTATION(#63849,#63882) ;
#63849=PRODUCT_DEFINITION_SHAPE('',$,#63899) ;
#63882=SHAPE_REPRESENTATION('',(#15892),#63812) ;
#63894=PRODUCT_DEFINITION_CONTEXT('part definition',#63944,'design') ;
#63899=PRODUCT_DEFINITION('Front_Plate','Front_Plate',#63915,#63894) ;
#63915=PRODUCT_DEFINITION_FORMATION('',$,#63950) ;
#63944=APPLICATION_CONTEXT(
'Core Data for Automotive Mechanical Design Process') ;
#63945=PRODUCT_CONTEXT('part definition',#63944,'mechanical') ;
#63950=PRODUCT('Front_Plate','Front_Plate',$,(#63945)) ;
#63963=PRESENTATION_STYLE_ASSIGNMENT((#63968)) ;
#63968=SURFACE_STYLE_USAGE(.BOTH.,#63973) ;
#63973=SURFACE_SIDE_STYLE('',(#63978)) ;
#63978=SURFACE_STYLE_FILL_AREA(#63983) ;
#63983=FILL_AREA_STYLE('Opaque(160,160,160)',(#63988)) ;
#63988=FILL_AREA_STYLE_COLOUR('Opaque(160,160,160)',#63993) ;
#63993=COLOUR_RGB('Opaque(160,160,160)', 0.09019608, 0.27058824, 0.51372549) ;
ENDSEC;
END-ISO-10303-21;
